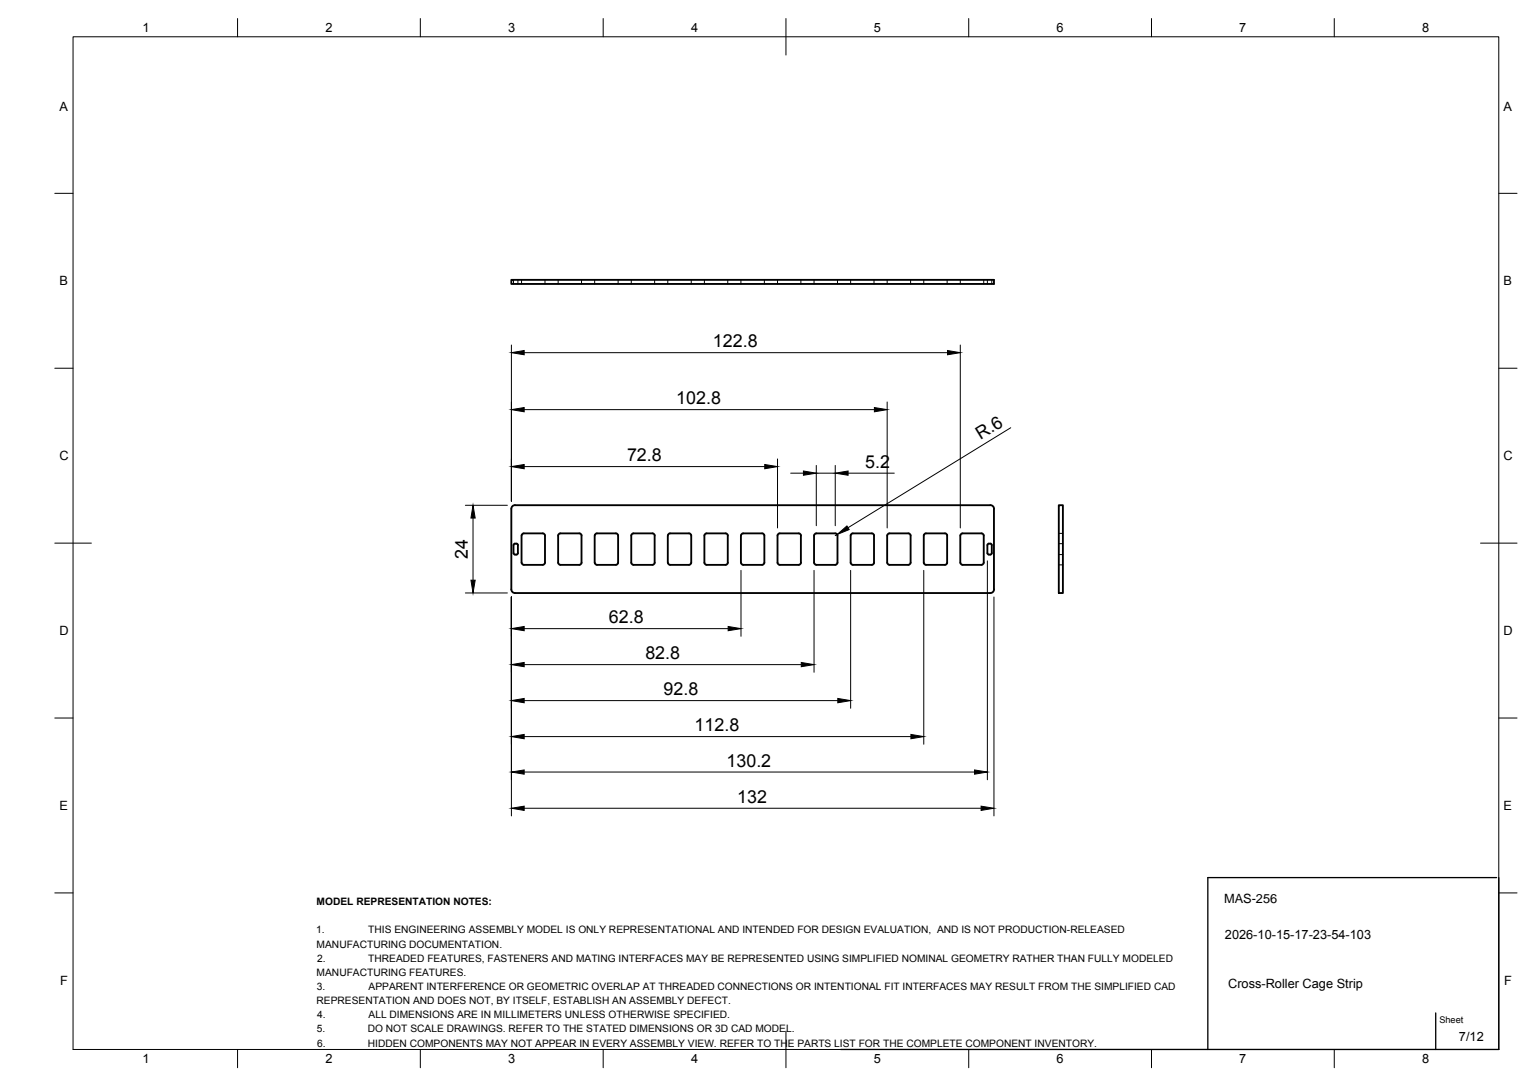
ISO-10303-21;
HEADER;
/* Generated by software containing ST-Developer
 * from STEP Tools, Inc. (www.steptools.com) 
 */

FILE_DESCRIPTION(
/* description */ (''),
/* implementation_level */ '2;1');

FILE_NAME(
/* name */ 'Cross-Roller Cage Strip.step',
/* time_stamp */ '2026-10-14T18:40:07-07:00',
/* author */ (''),
/* organization */ (''),
/* preprocessor_version */ 'ST-DEVELOPER v20.2',
/* originating_system */ 'Autodesk Translation Framework v15.15.0.0',
/* authorisation */ '');

FILE_SCHEMA (('AUTOMOTIVE_DESIGN { 1 0 10303 214 3 1 1 }'));
ENDSEC;

DATA;
#10=MECHANICAL_DESIGN_GEOMETRIC_PRESENTATION_REPRESENTATION('',(#835),#81040);
#815=SHAPE_REPRESENTATION_RELATIONSHIP('SRR','None',#81134,#825);
#825=ADVANCED_BREP_SHAPE_REPRESENTATION('',(#845),#81034);
#835=STYLED_ITEM('',(#81193),#845);
#845=MANIFOLD_SOLID_BREP('Body1',#15088);
#926=CYLINDRICAL_SURFACE('',#15818,0.400000000000027);
#927=CYLINDRICAL_SURFACE('',#15822,0.399999999999956);
#928=CYLINDRICAL_SURFACE('',#15826,0.399999999999945);
#929=CYLINDRICAL_SURFACE('',#15830,0.400000000000027);
#930=CYLINDRICAL_SURFACE('',#15834,0.399999999999996);
#931=CYLINDRICAL_SURFACE('',#15838,0.4);
#932=CYLINDRICAL_SURFACE('',#15842,0.399999999999996);
#933=CYLINDRICAL_SURFACE('',#15846,0.399999999999996);
#934=CYLINDRICAL_SURFACE('',#15850,0.600000000000005);
#935=CYLINDRICAL_SURFACE('',#15854,0.600000000000005);
#936=CYLINDRICAL_SURFACE('',#15858,0.600000000000005);
#937=CYLINDRICAL_SURFACE('',#15862,0.600000000000005);
#938=CYLINDRICAL_SURFACE('',#15866,0.600000000000005);
#939=CYLINDRICAL_SURFACE('',#15870,0.600000000000005);
#940=CYLINDRICAL_SURFACE('',#15874,0.600000000000005);
#941=CYLINDRICAL_SURFACE('',#15878,0.600000000000005);
#942=CYLINDRICAL_SURFACE('',#15882,0.599999999999987);
#943=CYLINDRICAL_SURFACE('',#15886,0.599999999999987);
#944=CYLINDRICAL_SURFACE('',#15890,0.599999999999987);
#945=CYLINDRICAL_SURFACE('',#15894,0.599999999999987);
#946=CYLINDRICAL_SURFACE('',#15898,0.599999999999987);
#947=CYLINDRICAL_SURFACE('',#15902,0.599999999999987);
#948=CYLINDRICAL_SURFACE('',#15906,0.599999999999987);
#949=CYLINDRICAL_SURFACE('',#15910,0.599999999999987);
#950=CYLINDRICAL_SURFACE('',#15914,0.599999999999987);
#951=CYLINDRICAL_SURFACE('',#15918,0.599999999999987);
#952=CYLINDRICAL_SURFACE('',#15922,0.599999999999987);
#953=CYLINDRICAL_SURFACE('',#15926,0.599999999999987);
#954=CYLINDRICAL_SURFACE('',#15930,0.600000000000001);
#955=CYLINDRICAL_SURFACE('',#15934,0.600000000000005);
#956=CYLINDRICAL_SURFACE('',#15938,0.599999999999998);
#957=CYLINDRICAL_SURFACE('',#15942,0.600000000000005);
#958=CYLINDRICAL_SURFACE('',#15946,0.600000000000001);
#959=CYLINDRICAL_SURFACE('',#15950,0.600000000000005);
#960=CYLINDRICAL_SURFACE('',#15954,0.600000000000003);
#961=CYLINDRICAL_SURFACE('',#15958,0.600000000000005);
#962=CYLINDRICAL_SURFACE('',#15962,0.599999999999996);
#963=CYLINDRICAL_SURFACE('',#15966,0.600000000000005);
#964=CYLINDRICAL_SURFACE('',#15970,0.599999999999998);
#965=CYLINDRICAL_SURFACE('',#15974,0.600000000000005);
#966=CYLINDRICAL_SURFACE('',#15978,0.599999999999987);
#967=CYLINDRICAL_SURFACE('',#15982,0.599999999999987);
#968=CYLINDRICAL_SURFACE('',#15986,0.599999999999987);
#969=CYLINDRICAL_SURFACE('',#15990,0.599999999999987);
#970=CYLINDRICAL_SURFACE('',#15994,0.600000000000001);
#971=CYLINDRICAL_SURFACE('',#15998,0.600000000000005);
#972=CYLINDRICAL_SURFACE('',#16002,0.600000000000003);
#973=CYLINDRICAL_SURFACE('',#16006,0.600000000000005);
#974=CYLINDRICAL_SURFACE('',#16010,0.599999999999987);
#975=CYLINDRICAL_SURFACE('',#16014,0.600000000000005);
#976=CYLINDRICAL_SURFACE('',#16018,0.600000000000005);
#977=CYLINDRICAL_SURFACE('',#16022,0.599999999999987);
#978=CYLINDRICAL_SURFACE('',#16026,0.600000000000005);
#979=CYLINDRICAL_SURFACE('',#16030,0.600000000000005);
#980=CYLINDRICAL_SURFACE('',#16034,0.600000000000005);
#981=CYLINDRICAL_SURFACE('',#16038,0.600000000000005);
#982=CYLINDRICAL_SURFACE('',#16042,0.600000000000027);
#983=CYLINDRICAL_SURFACE('',#16046,0.600000000000023);
#984=CYLINDRICAL_SURFACE('',#16050,0.600000000000025);
#985=CYLINDRICAL_SURFACE('',#16054,0.600000000000023);
#986=CYLINDRICAL_SURFACE('',#16058,1.);
#987=CYLINDRICAL_SURFACE('',#16062,1.00000000000001);
#988=CYLINDRICAL_SURFACE('',#16066,1.00000000000001);
#989=CYLINDRICAL_SURFACE('',#16070,1.);
#1176=FACE_BOUND('',#2884,.T.);
#1177=FACE_BOUND('',#2885,.T.);
#1178=FACE_BOUND('',#2886,.T.);
#1179=FACE_BOUND('',#2887,.T.);
#1180=FACE_BOUND('',#2888,.T.);
#1181=FACE_BOUND('',#2889,.T.);
#1182=FACE_BOUND('',#2890,.T.);
#1183=FACE_BOUND('',#2891,.T.);
#1184=FACE_BOUND('',#2892,.T.);
#1185=FACE_BOUND('',#2893,.T.);
#1186=FACE_BOUND('',#2894,.T.);
#1187=FACE_BOUND('',#2895,.T.);
#1188=FACE_BOUND('',#2896,.T.);
#1189=FACE_BOUND('',#2897,.T.);
#1190=FACE_BOUND('',#2898,.T.);
#1191=FACE_BOUND('',#2900,.T.);
#1192=FACE_BOUND('',#2901,.T.);
#1193=FACE_BOUND('',#2902,.T.);
#1194=FACE_BOUND('',#2903,.T.);
#1195=FACE_BOUND('',#2904,.T.);
#1196=FACE_BOUND('',#2905,.T.);
#1197=FACE_BOUND('',#2906,.T.);
#1198=FACE_BOUND('',#2907,.T.);
#1199=FACE_BOUND('',#2908,.T.);
#1200=FACE_BOUND('',#2909,.T.);
#1201=FACE_BOUND('',#2910,.T.);
#1202=FACE_BOUND('',#2911,.T.);
#1203=FACE_BOUND('',#2912,.T.);
#1204=FACE_BOUND('',#2913,.T.);
#1205=FACE_BOUND('',#2914,.T.);
#1362=PLANE('',#15817);
#1363=PLANE('',#15821);
#1364=PLANE('',#15825);
#1365=PLANE('',#15829);
#1366=PLANE('',#15833);
#1367=PLANE('',#15837);
#1368=PLANE('',#15841);
#1369=PLANE('',#15845);
#1370=PLANE('',#15849);
#1371=PLANE('',#15853);
#1372=PLANE('',#15857);
#1373=PLANE('',#15861);
#1374=PLANE('',#15865);
#1375=PLANE('',#15869);
#1376=PLANE('',#15873);
#1377=PLANE('',#15877);
#1378=PLANE('',#15881);
#1379=PLANE('',#15885);
#1380=PLANE('',#15889);
#1381=PLANE('',#15893);
#1382=PLANE('',#15897);
#1383=PLANE('',#15901);
#1384=PLANE('',#15905);
#1385=PLANE('',#15909);
#1386=PLANE('',#15913);
#1387=PLANE('',#15917);
#1388=PLANE('',#15921);
#1389=PLANE('',#15925);
#1390=PLANE('',#15929);
#1391=PLANE('',#15933);
#1392=PLANE('',#15937);
#1393=PLANE('',#15941);
#1394=PLANE('',#15945);
#1395=PLANE('',#15949);
#1396=PLANE('',#15953);
#1397=PLANE('',#15957);
#1398=PLANE('',#15961);
#1399=PLANE('',#15965);
#1400=PLANE('',#15969);
#1401=PLANE('',#15973);
#1402=PLANE('',#15977);
#1403=PLANE('',#15981);
#1404=PLANE('',#15985);
#1405=PLANE('',#15989);
#1406=PLANE('',#15993);
#1407=PLANE('',#15997);
#1408=PLANE('',#16001);
#1409=PLANE('',#16005);
#1410=PLANE('',#16009);
#1411=PLANE('',#16013);
#1412=PLANE('',#16017);
#1413=PLANE('',#16021);
#1414=PLANE('',#16025);
#1415=PLANE('',#16029);
#1416=PLANE('',#16033);
#1417=PLANE('',#16037);
#1418=PLANE('',#16041);
#1419=PLANE('',#16045);
#1420=PLANE('',#16049);
#1421=PLANE('',#16053);
#1422=PLANE('',#16057);
#1423=PLANE('',#16061);
#1424=PLANE('',#16065);
#1425=PLANE('',#16069);
#1426=PLANE('',#16073);
#1427=PLANE('',#16074);
#1919=FACE_OUTER_BOUND('',#2755,.T.);
#1920=FACE_OUTER_BOUND('',#2756,.T.);
#1921=FACE_OUTER_BOUND('',#2757,.T.);
#1922=FACE_OUTER_BOUND('',#2758,.T.);
#1923=FACE_OUTER_BOUND('',#2759,.T.);
#1924=FACE_OUTER_BOUND('',#2760,.T.);
#1925=FACE_OUTER_BOUND('',#2761,.T.);
#1926=FACE_OUTER_BOUND('',#2762,.T.);
#1927=FACE_OUTER_BOUND('',#2763,.T.);
#1928=FACE_OUTER_BOUND('',#2764,.T.);
#1929=FACE_OUTER_BOUND('',#2765,.T.);
#1930=FACE_OUTER_BOUND('',#2766,.T.);
#1931=FACE_OUTER_BOUND('',#2767,.T.);
#1932=FACE_OUTER_BOUND('',#2768,.T.);
#1933=FACE_OUTER_BOUND('',#2769,.T.);
#1934=FACE_OUTER_BOUND('',#2770,.T.);
#1935=FACE_OUTER_BOUND('',#2771,.T.);
#1936=FACE_OUTER_BOUND('',#2772,.T.);
#1937=FACE_OUTER_BOUND('',#2773,.T.);
#1938=FACE_OUTER_BOUND('',#2774,.T.);
#1939=FACE_OUTER_BOUND('',#2775,.T.);
#1940=FACE_OUTER_BOUND('',#2776,.T.);
#1941=FACE_OUTER_BOUND('',#2777,.T.);
#1942=FACE_OUTER_BOUND('',#2778,.T.);
#1943=FACE_OUTER_BOUND('',#2779,.T.);
#1944=FACE_OUTER_BOUND('',#2780,.T.);
#1945=FACE_OUTER_BOUND('',#2781,.T.);
#1946=FACE_OUTER_BOUND('',#2782,.T.);
#1947=FACE_OUTER_BOUND('',#2783,.T.);
#1948=FACE_OUTER_BOUND('',#2784,.T.);
#1949=FACE_OUTER_BOUND('',#2785,.T.);
#1950=FACE_OUTER_BOUND('',#2786,.T.);
#1951=FACE_OUTER_BOUND('',#2787,.T.);
#1952=FACE_OUTER_BOUND('',#2788,.T.);
#1953=FACE_OUTER_BOUND('',#2789,.T.);
#1954=FACE_OUTER_BOUND('',#2790,.T.);
#1955=FACE_OUTER_BOUND('',#2791,.T.);
#1956=FACE_OUTER_BOUND('',#2792,.T.);
#1957=FACE_OUTER_BOUND('',#2793,.T.);
#1958=FACE_OUTER_BOUND('',#2794,.T.);
#1959=FACE_OUTER_BOUND('',#2795,.T.);
#1960=FACE_OUTER_BOUND('',#2796,.T.);
#1961=FACE_OUTER_BOUND('',#2797,.T.);
#1962=FACE_OUTER_BOUND('',#2798,.T.);
#1963=FACE_OUTER_BOUND('',#2799,.T.);
#1964=FACE_OUTER_BOUND('',#2800,.T.);
#1965=FACE_OUTER_BOUND('',#2801,.T.);
#1966=FACE_OUTER_BOUND('',#2802,.T.);
#1967=FACE_OUTER_BOUND('',#2803,.T.);
#1968=FACE_OUTER_BOUND('',#2804,.T.);
#1969=FACE_OUTER_BOUND('',#2805,.T.);
#1970=FACE_OUTER_BOUND('',#2806,.T.);
#1971=FACE_OUTER_BOUND('',#2807,.T.);
#1972=FACE_OUTER_BOUND('',#2808,.T.);
#1973=FACE_OUTER_BOUND('',#2809,.T.);
#1974=FACE_OUTER_BOUND('',#2810,.T.);
#1975=FACE_OUTER_BOUND('',#2811,.T.);
#1976=FACE_OUTER_BOUND('',#2812,.T.);
#1977=FACE_OUTER_BOUND('',#2813,.T.);
#1978=FACE_OUTER_BOUND('',#2814,.T.);
#1979=FACE_OUTER_BOUND('',#2815,.T.);
#1980=FACE_OUTER_BOUND('',#2816,.T.);
#1981=FACE_OUTER_BOUND('',#2817,.T.);
#1982=FACE_OUTER_BOUND('',#2818,.T.);
#1983=FACE_OUTER_BOUND('',#2819,.T.);
#1984=FACE_OUTER_BOUND('',#2820,.T.);
#1985=FACE_OUTER_BOUND('',#2821,.T.);
#1986=FACE_OUTER_BOUND('',#2822,.T.);
#1987=FACE_OUTER_BOUND('',#2823,.T.);
#1988=FACE_OUTER_BOUND('',#2824,.T.);
#1989=FACE_OUTER_BOUND('',#2825,.T.);
#1990=FACE_OUTER_BOUND('',#2826,.T.);
#1991=FACE_OUTER_BOUND('',#2827,.T.);
#1992=FACE_OUTER_BOUND('',#2828,.T.);
#1993=FACE_OUTER_BOUND('',#2829,.T.);
#1994=FACE_OUTER_BOUND('',#2830,.T.);
#1995=FACE_OUTER_BOUND('',#2831,.T.);
#1996=FACE_OUTER_BOUND('',#2832,.T.);
#1997=FACE_OUTER_BOUND('',#2833,.T.);
#1998=FACE_OUTER_BOUND('',#2834,.T.);
#1999=FACE_OUTER_BOUND('',#2835,.T.);
#2000=FACE_OUTER_BOUND('',#2836,.T.);
#2001=FACE_OUTER_BOUND('',#2837,.T.);
#2002=FACE_OUTER_BOUND('',#2838,.T.);
#2003=FACE_OUTER_BOUND('',#2839,.T.);
#2004=FACE_OUTER_BOUND('',#2840,.T.);
#2005=FACE_OUTER_BOUND('',#2841,.T.);
#2006=FACE_OUTER_BOUND('',#2842,.T.);
#2007=FACE_OUTER_BOUND('',#2843,.T.);
#2008=FACE_OUTER_BOUND('',#2844,.T.);
#2009=FACE_OUTER_BOUND('',#2845,.T.);
#2010=FACE_OUTER_BOUND('',#2846,.T.);
#2011=FACE_OUTER_BOUND('',#2847,.T.);
#2012=FACE_OUTER_BOUND('',#2848,.T.);
#2013=FACE_OUTER_BOUND('',#2849,.T.);
#2014=FACE_OUTER_BOUND('',#2850,.T.);
#2015=FACE_OUTER_BOUND('',#2851,.T.);
#2016=FACE_OUTER_BOUND('',#2852,.T.);
#2017=FACE_OUTER_BOUND('',#2853,.T.);
#2018=FACE_OUTER_BOUND('',#2854,.T.);
#2019=FACE_OUTER_BOUND('',#2855,.T.);
#2020=FACE_OUTER_BOUND('',#2856,.T.);
#2021=FACE_OUTER_BOUND('',#2857,.T.);
#2022=FACE_OUTER_BOUND('',#2858,.T.);
#2023=FACE_OUTER_BOUND('',#2859,.T.);
#2024=FACE_OUTER_BOUND('',#2860,.T.);
#2025=FACE_OUTER_BOUND('',#2861,.T.);
#2026=FACE_OUTER_BOUND('',#2862,.T.);
#2027=FACE_OUTER_BOUND('',#2863,.T.);
#2028=FACE_OUTER_BOUND('',#2864,.T.);
#2029=FACE_OUTER_BOUND('',#2865,.T.);
#2030=FACE_OUTER_BOUND('',#2866,.T.);
#2031=FACE_OUTER_BOUND('',#2867,.T.);
#2032=FACE_OUTER_BOUND('',#2868,.T.);
#2033=FACE_OUTER_BOUND('',#2869,.T.);
#2034=FACE_OUTER_BOUND('',#2870,.T.);
#2035=FACE_OUTER_BOUND('',#2871,.T.);
#2036=FACE_OUTER_BOUND('',#2872,.T.);
#2037=FACE_OUTER_BOUND('',#2873,.T.);
#2038=FACE_OUTER_BOUND('',#2874,.T.);
#2039=FACE_OUTER_BOUND('',#2875,.T.);
#2040=FACE_OUTER_BOUND('',#2876,.T.);
#2041=FACE_OUTER_BOUND('',#2877,.T.);
#2042=FACE_OUTER_BOUND('',#2878,.T.);
#2043=FACE_OUTER_BOUND('',#2879,.T.);
#2044=FACE_OUTER_BOUND('',#2880,.T.);
#2045=FACE_OUTER_BOUND('',#2881,.T.);
#2046=FACE_OUTER_BOUND('',#2882,.T.);
#2047=FACE_OUTER_BOUND('',#2883,.T.);
#2048=FACE_OUTER_BOUND('',#2899,.T.);
#2755=EDGE_LOOP('',(#11400,#11401,#11402,#11403));
#2756=EDGE_LOOP('',(#11404,#11405,#11406,#11407));
#2757=EDGE_LOOP('',(#11408,#11409,#11410,#11411));
#2758=EDGE_LOOP('',(#11412,#11413,#11414,#11415));
#2759=EDGE_LOOP('',(#11416,#11417,#11418,#11419));
#2760=EDGE_LOOP('',(#11420,#11421,#11422,#11423));
#2761=EDGE_LOOP('',(#11424,#11425,#11426,#11427));
#2762=EDGE_LOOP('',(#11428,#11429,#11430,#11431));
#2763=EDGE_LOOP('',(#11432,#11433,#11434,#11435));
#2764=EDGE_LOOP('',(#11436,#11437,#11438,#11439));
#2765=EDGE_LOOP('',(#11440,#11441,#11442,#11443));
#2766=EDGE_LOOP('',(#11444,#11445,#11446,#11447));
#2767=EDGE_LOOP('',(#11448,#11449,#11450,#11451));
#2768=EDGE_LOOP('',(#11452,#11453,#11454,#11455));
#2769=EDGE_LOOP('',(#11456,#11457,#11458,#11459));
#2770=EDGE_LOOP('',(#11460,#11461,#11462,#11463));
#2771=EDGE_LOOP('',(#11464,#11465,#11466,#11467));
#2772=EDGE_LOOP('',(#11468,#11469,#11470,#11471));
#2773=EDGE_LOOP('',(#11472,#11473,#11474,#11475));
#2774=EDGE_LOOP('',(#11476,#11477,#11478,#11479));
#2775=EDGE_LOOP('',(#11480,#11481,#11482,#11483));
#2776=EDGE_LOOP('',(#11484,#11485,#11486,#11487));
#2777=EDGE_LOOP('',(#11488,#11489,#11490,#11491));
#2778=EDGE_LOOP('',(#11492,#11493,#11494,#11495));
#2779=EDGE_LOOP('',(#11496,#11497,#11498,#11499));
#2780=EDGE_LOOP('',(#11500,#11501,#11502,#11503));
#2781=EDGE_LOOP('',(#11504,#11505,#11506,#11507));
#2782=EDGE_LOOP('',(#11508,#11509,#11510,#11511));
#2783=EDGE_LOOP('',(#11512,#11513,#11514,#11515));
#2784=EDGE_LOOP('',(#11516,#11517,#11518,#11519));
#2785=EDGE_LOOP('',(#11520,#11521,#11522,#11523));
#2786=EDGE_LOOP('',(#11524,#11525,#11526,#11527));
#2787=EDGE_LOOP('',(#11528,#11529,#11530,#11531));
#2788=EDGE_LOOP('',(#11532,#11533,#11534,#11535));
#2789=EDGE_LOOP('',(#11536,#11537,#11538,#11539));
#2790=EDGE_LOOP('',(#11540,#11541,#11542,#11543));
#2791=EDGE_LOOP('',(#11544,#11545,#11546,#11547));
#2792=EDGE_LOOP('',(#11548,#11549,#11550,#11551));
#2793=EDGE_LOOP('',(#11552,#11553,#11554,#11555));
#2794=EDGE_LOOP('',(#11556,#11557,#11558,#11559));
#2795=EDGE_LOOP('',(#11560,#11561,#11562,#11563));
#2796=EDGE_LOOP('',(#11564,#11565,#11566,#11567));
#2797=EDGE_LOOP('',(#11568,#11569,#11570,#11571));
#2798=EDGE_LOOP('',(#11572,#11573,#11574,#11575));
#2799=EDGE_LOOP('',(#11576,#11577,#11578,#11579));
#2800=EDGE_LOOP('',(#11580,#11581,#11582,#11583));
#2801=EDGE_LOOP('',(#11584,#11585,#11586,#11587));
#2802=EDGE_LOOP('',(#11588,#11589,#11590,#11591));
#2803=EDGE_LOOP('',(#11592,#11593,#11594,#11595));
#2804=EDGE_LOOP('',(#11596,#11597,#11598,#11599));
#2805=EDGE_LOOP('',(#11600,#11601,#11602,#11603));
#2806=EDGE_LOOP('',(#11604,#11605,#11606,#11607));
#2807=EDGE_LOOP('',(#11608,#11609,#11610,#11611));
#2808=EDGE_LOOP('',(#11612,#11613,#11614,#11615));
#2809=EDGE_LOOP('',(#11616,#11617,#11618,#11619));
#2810=EDGE_LOOP('',(#11620,#11621,#11622,#11623));
#2811=EDGE_LOOP('',(#11624,#11625,#11626,#11627));
#2812=EDGE_LOOP('',(#11628,#11629,#11630,#11631));
#2813=EDGE_LOOP('',(#11632,#11633,#11634,#11635));
#2814=EDGE_LOOP('',(#11636,#11637,#11638,#11639));
#2815=EDGE_LOOP('',(#11640,#11641,#11642,#11643));
#2816=EDGE_LOOP('',(#11644,#11645,#11646,#11647));
#2817=EDGE_LOOP('',(#11648,#11649,#11650,#11651));
#2818=EDGE_LOOP('',(#11652,#11653,#11654,#11655));
#2819=EDGE_LOOP('',(#11656,#11657,#11658,#11659));
#2820=EDGE_LOOP('',(#11660,#11661,#11662,#11663));
#2821=EDGE_LOOP('',(#11664,#11665,#11666,#11667));
#2822=EDGE_LOOP('',(#11668,#11669,#11670,#11671));
#2823=EDGE_LOOP('',(#11672,#11673,#11674,#11675));
#2824=EDGE_LOOP('',(#11676,#11677,#11678,#11679));
#2825=EDGE_LOOP('',(#11680,#11681,#11682,#11683));
#2826=EDGE_LOOP('',(#11684,#11685,#11686,#11687));
#2827=EDGE_LOOP('',(#11688,#11689,#11690,#11691));
#2828=EDGE_LOOP('',(#11692,#11693,#11694,#11695));
#2829=EDGE_LOOP('',(#11696,#11697,#11698,#11699));
#2830=EDGE_LOOP('',(#11700,#11701,#11702,#11703));
#2831=EDGE_LOOP('',(#11704,#11705,#11706,#11707));
#2832=EDGE_LOOP('',(#11708,#11709,#11710,#11711));
#2833=EDGE_LOOP('',(#11712,#11713,#11714,#11715));
#2834=EDGE_LOOP('',(#11716,#11717,#11718,#11719));
#2835=EDGE_LOOP('',(#11720,#11721,#11722,#11723));
#2836=EDGE_LOOP('',(#11724,#11725,#11726,#11727));
#2837=EDGE_LOOP('',(#11728,#11729,#11730,#11731));
#2838=EDGE_LOOP('',(#11732,#11733,#11734,#11735));
#2839=EDGE_LOOP('',(#11736,#11737,#11738,#11739));
#2840=EDGE_LOOP('',(#11740,#11741,#11742,#11743));
#2841=EDGE_LOOP('',(#11744,#11745,#11746,#11747));
#2842=EDGE_LOOP('',(#11748,#11749,#11750,#11751));
#2843=EDGE_LOOP('',(#11752,#11753,#11754,#11755));
#2844=EDGE_LOOP('',(#11756,#11757,#11758,#11759));
#2845=EDGE_LOOP('',(#11760,#11761,#11762,#11763));
#2846=EDGE_LOOP('',(#11764,#11765,#11766,#11767));
#2847=EDGE_LOOP('',(#11768,#11769,#11770,#11771));
#2848=EDGE_LOOP('',(#11772,#11773,#11774,#11775));
#2849=EDGE_LOOP('',(#11776,#11777,#11778,#11779));
#2850=EDGE_LOOP('',(#11780,#11781,#11782,#11783));
#2851=EDGE_LOOP('',(#11784,#11785,#11786,#11787));
#2852=EDGE_LOOP('',(#11788,#11789,#11790,#11791));
#2853=EDGE_LOOP('',(#11792,#11793,#11794,#11795));
#2854=EDGE_LOOP('',(#11796,#11797,#11798,#11799));
#2855=EDGE_LOOP('',(#11800,#11801,#11802,#11803));
#2856=EDGE_LOOP('',(#11804,#11805,#11806,#11807));
#2857=EDGE_LOOP('',(#11808,#11809,#11810,#11811));
#2858=EDGE_LOOP('',(#11812,#11813,#11814,#11815));
#2859=EDGE_LOOP('',(#11816,#11817,#11818,#11819));
#2860=EDGE_LOOP('',(#11820,#11821,#11822,#11823));
#2861=EDGE_LOOP('',(#11824,#11825,#11826,#11827));
#2862=EDGE_LOOP('',(#11828,#11829,#11830,#11831));
#2863=EDGE_LOOP('',(#11832,#11833,#11834,#11835));
#2864=EDGE_LOOP('',(#11836,#11837,#11838,#11839));
#2865=EDGE_LOOP('',(#11840,#11841,#11842,#11843));
#2866=EDGE_LOOP('',(#11844,#11845,#11846,#11847));
#2867=EDGE_LOOP('',(#11848,#11849,#11850,#11851));
#2868=EDGE_LOOP('',(#11852,#11853,#11854,#11855));
#2869=EDGE_LOOP('',(#11856,#11857,#11858,#11859));
#2870=EDGE_LOOP('',(#11860,#11861,#11862,#11863));
#2871=EDGE_LOOP('',(#11864,#11865,#11866,#11867));
#2872=EDGE_LOOP('',(#11868,#11869,#11870,#11871));
#2873=EDGE_LOOP('',(#11872,#11873,#11874,#11875));
#2874=EDGE_LOOP('',(#11876,#11877,#11878,#11879));
#2875=EDGE_LOOP('',(#11880,#11881,#11882,#11883));
#2876=EDGE_LOOP('',(#11884,#11885,#11886,#11887));
#2877=EDGE_LOOP('',(#11888,#11889,#11890,#11891));
#2878=EDGE_LOOP('',(#11892,#11893,#11894,#11895));
#2879=EDGE_LOOP('',(#11896,#11897,#11898,#11899));
#2880=EDGE_LOOP('',(#11900,#11901,#11902,#11903));
#2881=EDGE_LOOP('',(#11904,#11905,#11906,#11907));
#2882=EDGE_LOOP('',(#11908,#11909,#11910,#11911));
#2883=EDGE_LOOP('',(#11912,#11913,#11914,#11915,#11916,#11917,#11918,#11919));
#2884=EDGE_LOOP('',(#11920,#11921,#11922,#11923,#11924,#11925,#11926,#11927));
#2885=EDGE_LOOP('',(#11928,#11929,#11930,#11931,#11932,#11933,#11934,#11935));
#2886=EDGE_LOOP('',(#11936,#11937,#11938,#11939,#11940,#11941,#11942,#11943));
#2887=EDGE_LOOP('',(#11944,#11945,#11946,#11947,#11948,#11949,#11950,#11951));
#2888=EDGE_LOOP('',(#11952,#11953,#11954,#11955,#11956,#11957,#11958,#11959));
#2889=EDGE_LOOP('',(#11960,#11961,#11962,#11963,#11964,#11965,#11966,#11967));
#2890=EDGE_LOOP('',(#11968,#11969,#11970,#11971,#11972,#11973,#11974,#11975));
#2891=EDGE_LOOP('',(#11976,#11977,#11978,#11979,#11980,#11981,#11982,#11983));
#2892=EDGE_LOOP('',(#11984,#11985,#11986,#11987,#11988,#11989,#11990,#11991));
#2893=EDGE_LOOP('',(#11992,#11993,#11994,#11995,#11996,#11997,#11998,#11999));
#2894=EDGE_LOOP('',(#12000,#12001,#12002,#12003,#12004,#12005,#12006,#12007));
#2895=EDGE_LOOP('',(#12008,#12009,#12010,#12011,#12012,#12013,#12014,#12015));
#2896=EDGE_LOOP('',(#12016,#12017,#12018,#12019,#12020,#12021,#12022,#12023));
#2897=EDGE_LOOP('',(#12024,#12025,#12026,#12027,#12028,#12029,#12030,#12031));
#2898=EDGE_LOOP('',(#12032,#12033,#12034,#12035,#12036,#12037,#12038,#12039));
#2899=EDGE_LOOP('',(#12040,#12041,#12042,#12043,#12044,#12045,#12046,#12047));
#2900=EDGE_LOOP('',(#12048,#12049,#12050,#12051,#12052,#12053,#12054,#12055));
#2901=EDGE_LOOP('',(#12056,#12057,#12058,#12059,#12060,#12061,#12062,#12063));
#2902=EDGE_LOOP('',(#12064,#12065,#12066,#12067,#12068,#12069,#12070,#12071));
#2903=EDGE_LOOP('',(#12072,#12073,#12074,#12075,#12076,#12077,#12078,#12079));
#2904=EDGE_LOOP('',(#12080,#12081,#12082,#12083,#12084,#12085,#12086,#12087));
#2905=EDGE_LOOP('',(#12088,#12089,#12090,#12091,#12092,#12093,#12094,#12095));
#2906=EDGE_LOOP('',(#12096,#12097,#12098,#12099,#12100,#12101,#12102,#12103));
#2907=EDGE_LOOP('',(#12104,#12105,#12106,#12107,#12108,#12109,#12110,#12111));
#2908=EDGE_LOOP('',(#12112,#12113,#12114,#12115,#12116,#12117,#12118,#12119));
#2909=EDGE_LOOP('',(#12120,#12121,#12122,#12123,#12124,#12125,#12126,#12127));
#2910=EDGE_LOOP('',(#12128,#12129,#12130,#12131,#12132,#12133,#12134,#12135));
#2911=EDGE_LOOP('',(#12136,#12137,#12138,#12139,#12140,#12141,#12142,#12143));
#2912=EDGE_LOOP('',(#12144,#12145,#12146,#12147,#12148,#12149,#12150,#12151));
#2913=EDGE_LOOP('',(#12152,#12153,#12154,#12155,#12156,#12157,#12158,#12159));
#2914=EDGE_LOOP('',(#12160,#12161,#12162,#12163,#12164,#12165,#12166,#12167));
#3730=LINE('',#22250,#4842);
#3731=LINE('',#22252,#4843);
#3732=LINE('',#22254,#4844);
#3733=LINE('',#22255,#4845);
#3734=LINE('',#22260,#4846);
#3735=LINE('',#22264,#4847);
#3736=LINE('',#22266,#4848);
#3737=LINE('',#22267,#4849);
#3738=LINE('',#22272,#4850);
#3739=LINE('',#22276,#4851);
#3740=LINE('',#22278,#4852);
#3741=LINE('',#22279,#4853);
#3742=LINE('',#22284,#4854);
#3743=LINE('',#22288,#4855);
#3744=LINE('',#22290,#4856);
#3745=LINE('',#22291,#4857);
#3746=LINE('',#22298,#4858);
#3747=LINE('',#22300,#4859);
#3748=LINE('',#22302,#4860);
#3749=LINE('',#22303,#4861);
#3750=LINE('',#22308,#4862);
#3751=LINE('',#22312,#4863);
#3752=LINE('',#22314,#4864);
#3753=LINE('',#22315,#4865);
#3754=LINE('',#22320,#4866);
#3755=LINE('',#22324,#4867);
#3756=LINE('',#22326,#4868);
#3757=LINE('',#22327,#4869);
#3758=LINE('',#22332,#4870);
#3759=LINE('',#22336,#4871);
#3760=LINE('',#22338,#4872);
#3761=LINE('',#22339,#4873);
#3762=LINE('',#22346,#4874);
#3763=LINE('',#22348,#4875);
#3764=LINE('',#22350,#4876);
#3765=LINE('',#22351,#4877);
#3766=LINE('',#22356,#4878);
#3767=LINE('',#22360,#4879);
#3768=LINE('',#22362,#4880);
#3769=LINE('',#22363,#4881);
#3770=LINE('',#22368,#4882);
#3771=LINE('',#22372,#4883);
#3772=LINE('',#22374,#4884);
#3773=LINE('',#22375,#4885);
#3774=LINE('',#22380,#4886);
#3775=LINE('',#22384,#4887);
#3776=LINE('',#22386,#4888);
#3777=LINE('',#22387,#4889);
#3778=LINE('',#22394,#4890);
#3779=LINE('',#22396,#4891);
#3780=LINE('',#22398,#4892);
#3781=LINE('',#22399,#4893);
#3782=LINE('',#22404,#4894);
#3783=LINE('',#22408,#4895);
#3784=LINE('',#22410,#4896);
#3785=LINE('',#22411,#4897);
#3786=LINE('',#22416,#4898);
#3787=LINE('',#22420,#4899);
#3788=LINE('',#22422,#4900);
#3789=LINE('',#22423,#4901);
#3790=LINE('',#22428,#4902);
#3791=LINE('',#22432,#4903);
#3792=LINE('',#22434,#4904);
#3793=LINE('',#22435,#4905);
#3794=LINE('',#22442,#4906);
#3795=LINE('',#22444,#4907);
#3796=LINE('',#22446,#4908);
#3797=LINE('',#22447,#4909);
#3798=LINE('',#22452,#4910);
#3799=LINE('',#22456,#4911);
#3800=LINE('',#22458,#4912);
#3801=LINE('',#22459,#4913);
#3802=LINE('',#22464,#4914);
#3803=LINE('',#22468,#4915);
#3804=LINE('',#22470,#4916);
#3805=LINE('',#22471,#4917);
#3806=LINE('',#22476,#4918);
#3807=LINE('',#22480,#4919);
#3808=LINE('',#22482,#4920);
#3809=LINE('',#22483,#4921);
#3810=LINE('',#22490,#4922);
#3811=LINE('',#22492,#4923);
#3812=LINE('',#22494,#4924);
#3813=LINE('',#22495,#4925);
#3814=LINE('',#22500,#4926);
#3815=LINE('',#22504,#4927);
#3816=LINE('',#22506,#4928);
#3817=LINE('',#22507,#4929);
#3818=LINE('',#22512,#4930);
#3819=LINE('',#22516,#4931);
#3820=LINE('',#22518,#4932);
#3821=LINE('',#22519,#4933);
#3822=LINE('',#22524,#4934);
#3823=LINE('',#22528,#4935);
#3824=LINE('',#22530,#4936);
#3825=LINE('',#22531,#4937);
#3826=LINE('',#22538,#4938);
#3827=LINE('',#22540,#4939);
#3828=LINE('',#22542,#4940);
#3829=LINE('',#22543,#4941);
#3830=LINE('',#22548,#4942);
#3831=LINE('',#22552,#4943);
#3832=LINE('',#22554,#4944);
#3833=LINE('',#22555,#4945);
#3834=LINE('',#22560,#4946);
#3835=LINE('',#22564,#4947);
#3836=LINE('',#22566,#4948);
#3837=LINE('',#22567,#4949);
#3838=LINE('',#22572,#4950);
#3839=LINE('',#22576,#4951);
#3840=LINE('',#22578,#4952);
#3841=LINE('',#22579,#4953);
#3842=LINE('',#22586,#4954);
#3843=LINE('',#22588,#4955);
#3844=LINE('',#22590,#4956);
#3845=LINE('',#22591,#4957);
#3846=LINE('',#22596,#4958);
#3847=LINE('',#22600,#4959);
#3848=LINE('',#22602,#4960);
#3849=LINE('',#22603,#4961);
#3850=LINE('',#22608,#4962);
#3851=LINE('',#22612,#4963);
#3852=LINE('',#22614,#4964);
#3853=LINE('',#22615,#4965);
#3854=LINE('',#22620,#4966);
#3855=LINE('',#22624,#4967);
#3856=LINE('',#22626,#4968);
#3857=LINE('',#22627,#4969);
#3858=LINE('',#22634,#4970);
#3859=LINE('',#22636,#4971);
#3860=LINE('',#22638,#4972);
#3861=LINE('',#22639,#4973);
#3862=LINE('',#22644,#4974);
#3863=LINE('',#22648,#4975);
#3864=LINE('',#22650,#4976);
#3865=LINE('',#22651,#4977);
#3866=LINE('',#22656,#4978);
#3867=LINE('',#22660,#4979);
#3868=LINE('',#22662,#4980);
#3869=LINE('',#22663,#4981);
#3870=LINE('',#22668,#4982);
#3871=LINE('',#22672,#4983);
#3872=LINE('',#22674,#4984);
#3873=LINE('',#22675,#4985);
#3874=LINE('',#22682,#4986);
#3875=LINE('',#22684,#4987);
#3876=LINE('',#22686,#4988);
#3877=LINE('',#22687,#4989);
#3878=LINE('',#22692,#4990);
#3879=LINE('',#22696,#4991);
#3880=LINE('',#22698,#4992);
#3881=LINE('',#22699,#4993);
#3882=LINE('',#22704,#4994);
#3883=LINE('',#22708,#4995);
#3884=LINE('',#22710,#4996);
#3885=LINE('',#22711,#4997);
#3886=LINE('',#22716,#4998);
#3887=LINE('',#22720,#4999);
#3888=LINE('',#22722,#5000);
#3889=LINE('',#22723,#5001);
#3890=LINE('',#22730,#5002);
#3891=LINE('',#22732,#5003);
#3892=LINE('',#22734,#5004);
#3893=LINE('',#22735,#5005);
#3894=LINE('',#22740,#5006);
#3895=LINE('',#22744,#5007);
#3896=LINE('',#22746,#5008);
#3897=LINE('',#22747,#5009);
#3898=LINE('',#22752,#5010);
#3899=LINE('',#22756,#5011);
#3900=LINE('',#22758,#5012);
#3901=LINE('',#22759,#5013);
#3902=LINE('',#22764,#5014);
#3903=LINE('',#22768,#5015);
#3904=LINE('',#22770,#5016);
#3905=LINE('',#22771,#5017);
#3906=LINE('',#22778,#5018);
#3907=LINE('',#22780,#5019);
#3908=LINE('',#22782,#5020);
#3909=LINE('',#22783,#5021);
#3910=LINE('',#22788,#5022);
#3911=LINE('',#22792,#5023);
#3912=LINE('',#22794,#5024);
#3913=LINE('',#22795,#5025);
#3914=LINE('',#22800,#5026);
#3915=LINE('',#22804,#5027);
#3916=LINE('',#22806,#5028);
#3917=LINE('',#22807,#5029);
#3918=LINE('',#22812,#5030);
#3919=LINE('',#22816,#5031);
#3920=LINE('',#22818,#5032);
#3921=LINE('',#22819,#5033);
#3922=LINE('',#22826,#5034);
#3923=LINE('',#22828,#5035);
#3924=LINE('',#22830,#5036);
#3925=LINE('',#22831,#5037);
#3926=LINE('',#22836,#5038);
#3927=LINE('',#22840,#5039);
#3928=LINE('',#22842,#5040);
#3929=LINE('',#22843,#5041);
#3930=LINE('',#22848,#5042);
#3931=LINE('',#22852,#5043);
#3932=LINE('',#22854,#5044);
#3933=LINE('',#22855,#5045);
#3934=LINE('',#22860,#5046);
#3935=LINE('',#22864,#5047);
#3936=LINE('',#22866,#5048);
#3937=LINE('',#22867,#5049);
#3938=LINE('',#22874,#5050);
#3939=LINE('',#22876,#5051);
#3940=LINE('',#22878,#5052);
#3941=LINE('',#22879,#5053);
#3942=LINE('',#22884,#5054);
#3943=LINE('',#22888,#5055);
#3944=LINE('',#22890,#5056);
#3945=LINE('',#22891,#5057);
#3946=LINE('',#22896,#5058);
#3947=LINE('',#22900,#5059);
#3948=LINE('',#22902,#5060);
#3949=LINE('',#22903,#5061);
#3950=LINE('',#22908,#5062);
#3951=LINE('',#22912,#5063);
#3952=LINE('',#22914,#5064);
#3953=LINE('',#22915,#5065);
#3954=LINE('',#22922,#5066);
#3955=LINE('',#22924,#5067);
#3956=LINE('',#22926,#5068);
#3957=LINE('',#22927,#5069);
#3958=LINE('',#22932,#5070);
#3959=LINE('',#22936,#5071);
#3960=LINE('',#22938,#5072);
#3961=LINE('',#22939,#5073);
#3962=LINE('',#22944,#5074);
#3963=LINE('',#22948,#5075);
#3964=LINE('',#22950,#5076);
#3965=LINE('',#22951,#5077);
#3966=LINE('',#22956,#5078);
#3967=LINE('',#22960,#5079);
#3968=LINE('',#22962,#5080);
#3969=LINE('',#22963,#5081);
#3970=LINE('',#22970,#5082);
#3971=LINE('',#22972,#5083);
#3972=LINE('',#22974,#5084);
#3973=LINE('',#22975,#5085);
#3974=LINE('',#22981,#5086);
#3975=LINE('',#22984,#5087);
#3976=LINE('',#22986,#5088);
#3977=LINE('',#22987,#5089);
#3978=LINE('',#22993,#5090);
#3979=LINE('',#22996,#5091);
#3980=LINE('',#22998,#5092);
#3981=LINE('',#22999,#5093);
#3982=LINE('',#23005,#5094);
#3983=LINE('',#23008,#5095);
#3984=LINE('',#23010,#5096);
#3985=LINE('',#23011,#5097);
#4842=VECTOR('',#18356,10.);
#4843=VECTOR('',#18357,10.);
#4844=VECTOR('',#18358,10.);
#4845=VECTOR('',#18359,10.);
#4846=VECTOR('',#18364,10.);
#4847=VECTOR('',#18369,10.);
#4848=VECTOR('',#18370,10.);
#4849=VECTOR('',#18371,10.);
#4850=VECTOR('',#18376,10.);
#4851=VECTOR('',#18381,10.);
#4852=VECTOR('',#18382,10.);
#4853=VECTOR('',#18383,10.);
#4854=VECTOR('',#18388,10.);
#4855=VECTOR('',#18393,10.);
#4856=VECTOR('',#18394,10.);
#4857=VECTOR('',#18395,10.);
#4858=VECTOR('',#18404,10.);
#4859=VECTOR('',#18405,10.);
#4860=VECTOR('',#18406,10.);
#4861=VECTOR('',#18407,10.);
#4862=VECTOR('',#18412,10.);
#4863=VECTOR('',#18417,10.);
#4864=VECTOR('',#18418,10.);
#4865=VECTOR('',#18419,10.);
#4866=VECTOR('',#18424,10.);
#4867=VECTOR('',#18429,10.);
#4868=VECTOR('',#18430,10.);
#4869=VECTOR('',#18431,10.);
#4870=VECTOR('',#18436,10.);
#4871=VECTOR('',#18441,10.);
#4872=VECTOR('',#18442,10.);
#4873=VECTOR('',#18443,10.);
#4874=VECTOR('',#18452,10.);
#4875=VECTOR('',#18453,10.);
#4876=VECTOR('',#18454,10.);
#4877=VECTOR('',#18455,10.);
#4878=VECTOR('',#18460,10.);
#4879=VECTOR('',#18465,10.);
#4880=VECTOR('',#18466,10.);
#4881=VECTOR('',#18467,10.);
#4882=VECTOR('',#18472,10.);
#4883=VECTOR('',#18477,10.);
#4884=VECTOR('',#18478,10.);
#4885=VECTOR('',#18479,10.);
#4886=VECTOR('',#18484,10.);
#4887=VECTOR('',#18489,10.);
#4888=VECTOR('',#18490,10.);
#4889=VECTOR('',#18491,10.);
#4890=VECTOR('',#18500,10.);
#4891=VECTOR('',#18501,10.);
#4892=VECTOR('',#18502,10.);
#4893=VECTOR('',#18503,10.);
#4894=VECTOR('',#18508,10.);
#4895=VECTOR('',#18513,10.);
#4896=VECTOR('',#18514,10.);
#4897=VECTOR('',#18515,10.);
#4898=VECTOR('',#18520,10.);
#4899=VECTOR('',#18525,10.);
#4900=VECTOR('',#18526,10.);
#4901=VECTOR('',#18527,10.);
#4902=VECTOR('',#18532,10.);
#4903=VECTOR('',#18537,10.);
#4904=VECTOR('',#18538,10.);
#4905=VECTOR('',#18539,10.);
#4906=VECTOR('',#18548,10.);
#4907=VECTOR('',#18549,10.);
#4908=VECTOR('',#18550,10.);
#4909=VECTOR('',#18551,10.);
#4910=VECTOR('',#18556,10.);
#4911=VECTOR('',#18561,10.);
#4912=VECTOR('',#18562,10.);
#4913=VECTOR('',#18563,10.);
#4914=VECTOR('',#18568,10.);
#4915=VECTOR('',#18573,10.);
#4916=VECTOR('',#18574,10.);
#4917=VECTOR('',#18575,10.);
#4918=VECTOR('',#18580,10.);
#4919=VECTOR('',#18585,10.);
#4920=VECTOR('',#18586,10.);
#4921=VECTOR('',#18587,10.);
#4922=VECTOR('',#18596,10.);
#4923=VECTOR('',#18597,10.);
#4924=VECTOR('',#18598,10.);
#4925=VECTOR('',#18599,10.);
#4926=VECTOR('',#18604,10.);
#4927=VECTOR('',#18609,10.);
#4928=VECTOR('',#18610,10.);
#4929=VECTOR('',#18611,10.);
#4930=VECTOR('',#18616,10.);
#4931=VECTOR('',#18621,10.);
#4932=VECTOR('',#18622,10.);
#4933=VECTOR('',#18623,10.);
#4934=VECTOR('',#18628,10.);
#4935=VECTOR('',#18633,10.);
#4936=VECTOR('',#18634,10.);
#4937=VECTOR('',#18635,10.);
#4938=VECTOR('',#18644,10.);
#4939=VECTOR('',#18645,10.);
#4940=VECTOR('',#18646,10.);
#4941=VECTOR('',#18647,10.);
#4942=VECTOR('',#18652,10.);
#4943=VECTOR('',#18657,10.);
#4944=VECTOR('',#18658,10.);
#4945=VECTOR('',#18659,10.);
#4946=VECTOR('',#18664,10.);
#4947=VECTOR('',#18669,10.);
#4948=VECTOR('',#18670,10.);
#4949=VECTOR('',#18671,10.);
#4950=VECTOR('',#18676,10.);
#4951=VECTOR('',#18681,10.);
#4952=VECTOR('',#18682,10.);
#4953=VECTOR('',#18683,10.);
#4954=VECTOR('',#18692,10.);
#4955=VECTOR('',#18693,10.);
#4956=VECTOR('',#18694,10.);
#4957=VECTOR('',#18695,10.);
#4958=VECTOR('',#18700,10.);
#4959=VECTOR('',#18705,10.);
#4960=VECTOR('',#18706,10.);
#4961=VECTOR('',#18707,10.);
#4962=VECTOR('',#18712,10.);
#4963=VECTOR('',#18717,10.);
#4964=VECTOR('',#18718,10.);
#4965=VECTOR('',#18719,10.);
#4966=VECTOR('',#18724,10.);
#4967=VECTOR('',#18729,10.);
#4968=VECTOR('',#18730,10.);
#4969=VECTOR('',#18731,10.);
#4970=VECTOR('',#18740,10.);
#4971=VECTOR('',#18741,10.);
#4972=VECTOR('',#18742,10.);
#4973=VECTOR('',#18743,10.);
#4974=VECTOR('',#18748,10.);
#4975=VECTOR('',#18753,10.);
#4976=VECTOR('',#18754,10.);
#4977=VECTOR('',#18755,10.);
#4978=VECTOR('',#18760,10.);
#4979=VECTOR('',#18765,10.);
#4980=VECTOR('',#18766,10.);
#4981=VECTOR('',#18767,10.);
#4982=VECTOR('',#18772,10.);
#4983=VECTOR('',#18777,10.);
#4984=VECTOR('',#18778,10.);
#4985=VECTOR('',#18779,10.);
#4986=VECTOR('',#18788,10.);
#4987=VECTOR('',#18789,10.);
#4988=VECTOR('',#18790,10.);
#4989=VECTOR('',#18791,10.);
#4990=VECTOR('',#18796,10.);
#4991=VECTOR('',#18801,10.);
#4992=VECTOR('',#18802,10.);
#4993=VECTOR('',#18803,10.);
#4994=VECTOR('',#18808,10.);
#4995=VECTOR('',#18813,10.);
#4996=VECTOR('',#18814,10.);
#4997=VECTOR('',#18815,10.);
#4998=VECTOR('',#18820,10.);
#4999=VECTOR('',#18825,10.);
#5000=VECTOR('',#18826,10.);
#5001=VECTOR('',#18827,10.);
#5002=VECTOR('',#18836,10.);
#5003=VECTOR('',#18837,10.);
#5004=VECTOR('',#18838,10.);
#5005=VECTOR('',#18839,10.);
#5006=VECTOR('',#18844,10.);
#5007=VECTOR('',#18849,10.);
#5008=VECTOR('',#18850,10.);
#5009=VECTOR('',#18851,10.);
#5010=VECTOR('',#18856,10.);
#5011=VECTOR('',#18861,10.);
#5012=VECTOR('',#18862,10.);
#5013=VECTOR('',#18863,10.);
#5014=VECTOR('',#18868,10.);
#5015=VECTOR('',#18873,10.);
#5016=VECTOR('',#18874,10.);
#5017=VECTOR('',#18875,10.);
#5018=VECTOR('',#18884,10.);
#5019=VECTOR('',#18885,10.);
#5020=VECTOR('',#18886,10.);
#5021=VECTOR('',#18887,10.);
#5022=VECTOR('',#18892,10.);
#5023=VECTOR('',#18897,10.);
#5024=VECTOR('',#18898,10.);
#5025=VECTOR('',#18899,10.);
#5026=VECTOR('',#18904,10.);
#5027=VECTOR('',#18909,10.);
#5028=VECTOR('',#18910,10.);
#5029=VECTOR('',#18911,10.);
#5030=VECTOR('',#18916,10.);
#5031=VECTOR('',#18921,10.);
#5032=VECTOR('',#18922,10.);
#5033=VECTOR('',#18923,10.);
#5034=VECTOR('',#18932,10.);
#5035=VECTOR('',#18933,10.);
#5036=VECTOR('',#18934,10.);
#5037=VECTOR('',#18935,10.);
#5038=VECTOR('',#18940,10.);
#5039=VECTOR('',#18945,10.);
#5040=VECTOR('',#18946,10.);
#5041=VECTOR('',#18947,10.);
#5042=VECTOR('',#18952,10.);
#5043=VECTOR('',#18957,10.);
#5044=VECTOR('',#18958,10.);
#5045=VECTOR('',#18959,10.);
#5046=VECTOR('',#18964,10.);
#5047=VECTOR('',#18969,10.);
#5048=VECTOR('',#18970,10.);
#5049=VECTOR('',#18971,10.);
#5050=VECTOR('',#18980,10.);
#5051=VECTOR('',#18981,10.);
#5052=VECTOR('',#18982,10.);
#5053=VECTOR('',#18983,10.);
#5054=VECTOR('',#18988,10.);
#5055=VECTOR('',#18993,10.);
#5056=VECTOR('',#18994,10.);
#5057=VECTOR('',#18995,10.);
#5058=VECTOR('',#19000,10.);
#5059=VECTOR('',#19005,10.);
#5060=VECTOR('',#19006,10.);
#5061=VECTOR('',#19007,10.);
#5062=VECTOR('',#19012,10.);
#5063=VECTOR('',#19017,10.);
#5064=VECTOR('',#19018,10.);
#5065=VECTOR('',#19019,10.);
#5066=VECTOR('',#19028,10.);
#5067=VECTOR('',#19029,10.);
#5068=VECTOR('',#19030,10.);
#5069=VECTOR('',#19031,10.);
#5070=VECTOR('',#19036,10.);
#5071=VECTOR('',#19041,10.);
#5072=VECTOR('',#19042,10.);
#5073=VECTOR('',#19043,10.);
#5074=VECTOR('',#19048,10.);
#5075=VECTOR('',#19053,10.);
#5076=VECTOR('',#19054,10.);
#5077=VECTOR('',#19055,10.);
#5078=VECTOR('',#19060,10.);
#5079=VECTOR('',#19065,10.);
#5080=VECTOR('',#19066,10.);
#5081=VECTOR('',#19067,10.);
#5082=VECTOR('',#19076,10.);
#5083=VECTOR('',#19077,10.);
#5084=VECTOR('',#19078,10.);
#5085=VECTOR('',#19079,10.);
#5086=VECTOR('',#19086,10.);
#5087=VECTOR('',#19089,10.);
#5088=VECTOR('',#19090,10.);
#5089=VECTOR('',#19091,10.);
#5090=VECTOR('',#19098,10.);
#5091=VECTOR('',#19101,10.);
#5092=VECTOR('',#19102,10.);
#5093=VECTOR('',#19103,10.);
#5094=VECTOR('',#19110,10.);
#5095=VECTOR('',#19113,10.);
#5096=VECTOR('',#19114,10.);
#5097=VECTOR('',#19115,10.);
#5709=CIRCLE('',#15819,0.400000000000027);
#5710=CIRCLE('',#15820,0.400000000000027);
#5711=CIRCLE('',#15823,0.399999999999956);
#5712=CIRCLE('',#15824,0.399999999999956);
#5713=CIRCLE('',#15827,0.399999999999945);
#5714=CIRCLE('',#15828,0.399999999999945);
#5715=CIRCLE('',#15831,0.400000000000027);
#5716=CIRCLE('',#15832,0.400000000000027);
#5717=CIRCLE('',#15835,0.399999999999996);
#5718=CIRCLE('',#15836,0.399999999999996);
#5719=CIRCLE('',#15839,0.4);
#5720=CIRCLE('',#15840,0.4);
#5721=CIRCLE('',#15843,0.399999999999996);
#5722=CIRCLE('',#15844,0.399999999999996);
#5723=CIRCLE('',#15847,0.399999999999996);
#5724=CIRCLE('',#15848,0.399999999999996);
#5725=CIRCLE('',#15851,0.600000000000005);
#5726=CIRCLE('',#15852,0.600000000000005);
#5727=CIRCLE('',#15855,0.600000000000005);
#5728=CIRCLE('',#15856,0.600000000000005);
#5729=CIRCLE('',#15859,0.600000000000005);
#5730=CIRCLE('',#15860,0.600000000000005);
#5731=CIRCLE('',#15863,0.600000000000005);
#5732=CIRCLE('',#15864,0.600000000000005);
#5733=CIRCLE('',#15867,0.600000000000005);
#5734=CIRCLE('',#15868,0.600000000000005);
#5735=CIRCLE('',#15871,0.600000000000005);
#5736=CIRCLE('',#15872,0.600000000000005);
#5737=CIRCLE('',#15875,0.600000000000005);
#5738=CIRCLE('',#15876,0.600000000000005);
#5739=CIRCLE('',#15879,0.600000000000005);
#5740=CIRCLE('',#15880,0.600000000000005);
#5741=CIRCLE('',#15883,0.599999999999987);
#5742=CIRCLE('',#15884,0.599999999999987);
#5743=CIRCLE('',#15887,0.599999999999987);
#5744=CIRCLE('',#15888,0.599999999999987);
#5745=CIRCLE('',#15891,0.599999999999987);
#5746=CIRCLE('',#15892,0.599999999999987);
#5747=CIRCLE('',#15895,0.599999999999987);
#5748=CIRCLE('',#15896,0.599999999999987);
#5749=CIRCLE('',#15899,0.599999999999987);
#5750=CIRCLE('',#15900,0.599999999999987);
#5751=CIRCLE('',#15903,0.599999999999987);
#5752=CIRCLE('',#15904,0.599999999999987);
#5753=CIRCLE('',#15907,0.599999999999987);
#5754=CIRCLE('',#15908,0.599999999999987);
#5755=CIRCLE('',#15911,0.599999999999987);
#5756=CIRCLE('',#15912,0.599999999999987);
#5757=CIRCLE('',#15915,0.599999999999987);
#5758=CIRCLE('',#15916,0.599999999999987);
#5759=CIRCLE('',#15919,0.599999999999987);
#5760=CIRCLE('',#15920,0.599999999999987);
#5761=CIRCLE('',#15923,0.599999999999987);
#5762=CIRCLE('',#15924,0.599999999999987);
#5763=CIRCLE('',#15927,0.599999999999987);
#5764=CIRCLE('',#15928,0.599999999999987);
#5765=CIRCLE('',#15931,0.600000000000001);
#5766=CIRCLE('',#15932,0.600000000000001);
#5767=CIRCLE('',#15935,0.600000000000005);
#5768=CIRCLE('',#15936,0.600000000000005);
#5769=CIRCLE('',#15939,0.599999999999998);
#5770=CIRCLE('',#15940,0.599999999999998);
#5771=CIRCLE('',#15943,0.600000000000005);
#5772=CIRCLE('',#15944,0.600000000000005);
#5773=CIRCLE('',#15947,0.600000000000001);
#5774=CIRCLE('',#15948,0.600000000000001);
#5775=CIRCLE('',#15951,0.600000000000005);
#5776=CIRCLE('',#15952,0.600000000000005);
#5777=CIRCLE('',#15955,0.600000000000003);
#5778=CIRCLE('',#15956,0.600000000000003);
#5779=CIRCLE('',#15959,0.600000000000005);
#5780=CIRCLE('',#15960,0.600000000000005);
#5781=CIRCLE('',#15963,0.599999999999996);
#5782=CIRCLE('',#15964,0.599999999999996);
#5783=CIRCLE('',#15967,0.600000000000005);
#5784=CIRCLE('',#15968,0.600000000000005);
#5785=CIRCLE('',#15971,0.599999999999998);
#5786=CIRCLE('',#15972,0.599999999999998);
#5787=CIRCLE('',#15975,0.600000000000005);
#5788=CIRCLE('',#15976,0.600000000000005);
#5789=CIRCLE('',#15979,0.599999999999987);
#5790=CIRCLE('',#15980,0.599999999999987);
#5791=CIRCLE('',#15983,0.599999999999987);
#5792=CIRCLE('',#15984,0.599999999999987);
#5793=CIRCLE('',#15987,0.599999999999987);
#5794=CIRCLE('',#15988,0.599999999999987);
#5795=CIRCLE('',#15991,0.599999999999987);
#5796=CIRCLE('',#15992,0.599999999999987);
#5797=CIRCLE('',#15995,0.600000000000001);
#5798=CIRCLE('',#15996,0.600000000000001);
#5799=CIRCLE('',#15999,0.600000000000005);
#5800=CIRCLE('',#16000,0.600000000000005);
#5801=CIRCLE('',#16003,0.600000000000003);
#5802=CIRCLE('',#16004,0.600000000000003);
#5803=CIRCLE('',#16007,0.600000000000005);
#5804=CIRCLE('',#16008,0.600000000000005);
#5805=CIRCLE('',#16011,0.599999999999987);
#5806=CIRCLE('',#16012,0.599999999999987);
#5807=CIRCLE('',#16015,0.600000000000005);
#5808=CIRCLE('',#16016,0.600000000000005);
#5809=CIRCLE('',#16019,0.600000000000005);
#5810=CIRCLE('',#16020,0.600000000000005);
#5811=CIRCLE('',#16023,0.599999999999987);
#5812=CIRCLE('',#16024,0.599999999999987);
#5813=CIRCLE('',#16027,0.600000000000005);
#5814=CIRCLE('',#16028,0.600000000000005);
#5815=CIRCLE('',#16031,0.600000000000005);
#5816=CIRCLE('',#16032,0.600000000000005);
#5817=CIRCLE('',#16035,0.600000000000005);
#5818=CIRCLE('',#16036,0.600000000000005);
#5819=CIRCLE('',#16039,0.600000000000005);
#5820=CIRCLE('',#16040,0.600000000000005);
#5821=CIRCLE('',#16043,0.600000000000027);
#5822=CIRCLE('',#16044,0.600000000000027);
#5823=CIRCLE('',#16047,0.600000000000023);
#5824=CIRCLE('',#16048,0.600000000000023);
#5825=CIRCLE('',#16051,0.600000000000025);
#5826=CIRCLE('',#16052,0.600000000000025);
#5827=CIRCLE('',#16055,0.600000000000023);
#5828=CIRCLE('',#16056,0.600000000000023);
#5829=CIRCLE('',#16059,1.);
#5830=CIRCLE('',#16060,1.);
#5831=CIRCLE('',#16063,1.00000000000001);
#5832=CIRCLE('',#16064,1.00000000000001);
#5833=CIRCLE('',#16067,1.00000000000001);
#5834=CIRCLE('',#16068,1.00000000000001);
#5835=CIRCLE('',#16071,1.);
#5836=CIRCLE('',#16072,1.);
#6548=VERTEX_POINT('',#22248);
#6549=VERTEX_POINT('',#22249);
#6550=VERTEX_POINT('',#22251);
#6551=VERTEX_POINT('',#22253);
#6552=VERTEX_POINT('',#22257);
#6553=VERTEX_POINT('',#22259);
#6554=VERTEX_POINT('',#22263);
#6555=VERTEX_POINT('',#22265);
#6556=VERTEX_POINT('',#22269);
#6557=VERTEX_POINT('',#22271);
#6558=VERTEX_POINT('',#22275);
#6559=VERTEX_POINT('',#22277);
#6560=VERTEX_POINT('',#22281);
#6561=VERTEX_POINT('',#22283);
#6562=VERTEX_POINT('',#22287);
#6563=VERTEX_POINT('',#22289);
#6564=VERTEX_POINT('',#22296);
#6565=VERTEX_POINT('',#22297);
#6566=VERTEX_POINT('',#22299);
#6567=VERTEX_POINT('',#22301);
#6568=VERTEX_POINT('',#22305);
#6569=VERTEX_POINT('',#22307);
#6570=VERTEX_POINT('',#22311);
#6571=VERTEX_POINT('',#22313);
#6572=VERTEX_POINT('',#22317);
#6573=VERTEX_POINT('',#22319);
#6574=VERTEX_POINT('',#22323);
#6575=VERTEX_POINT('',#22325);
#6576=VERTEX_POINT('',#22329);
#6577=VERTEX_POINT('',#22331);
#6578=VERTEX_POINT('',#22335);
#6579=VERTEX_POINT('',#22337);
#6580=VERTEX_POINT('',#22344);
#6581=VERTEX_POINT('',#22345);
#6582=VERTEX_POINT('',#22347);
#6583=VERTEX_POINT('',#22349);
#6584=VERTEX_POINT('',#22353);
#6585=VERTEX_POINT('',#22355);
#6586=VERTEX_POINT('',#22359);
#6587=VERTEX_POINT('',#22361);
#6588=VERTEX_POINT('',#22365);
#6589=VERTEX_POINT('',#22367);
#6590=VERTEX_POINT('',#22371);
#6591=VERTEX_POINT('',#22373);
#6592=VERTEX_POINT('',#22377);
#6593=VERTEX_POINT('',#22379);
#6594=VERTEX_POINT('',#22383);
#6595=VERTEX_POINT('',#22385);
#6596=VERTEX_POINT('',#22392);
#6597=VERTEX_POINT('',#22393);
#6598=VERTEX_POINT('',#22395);
#6599=VERTEX_POINT('',#22397);
#6600=VERTEX_POINT('',#22401);
#6601=VERTEX_POINT('',#22403);
#6602=VERTEX_POINT('',#22407);
#6603=VERTEX_POINT('',#22409);
#6604=VERTEX_POINT('',#22413);
#6605=VERTEX_POINT('',#22415);
#6606=VERTEX_POINT('',#22419);
#6607=VERTEX_POINT('',#22421);
#6608=VERTEX_POINT('',#22425);
#6609=VERTEX_POINT('',#22427);
#6610=VERTEX_POINT('',#22431);
#6611=VERTEX_POINT('',#22433);
#6612=VERTEX_POINT('',#22440);
#6613=VERTEX_POINT('',#22441);
#6614=VERTEX_POINT('',#22443);
#6615=VERTEX_POINT('',#22445);
#6616=VERTEX_POINT('',#22449);
#6617=VERTEX_POINT('',#22451);
#6618=VERTEX_POINT('',#22455);
#6619=VERTEX_POINT('',#22457);
#6620=VERTEX_POINT('',#22461);
#6621=VERTEX_POINT('',#22463);
#6622=VERTEX_POINT('',#22467);
#6623=VERTEX_POINT('',#22469);
#6624=VERTEX_POINT('',#22473);
#6625=VERTEX_POINT('',#22475);
#6626=VERTEX_POINT('',#22479);
#6627=VERTEX_POINT('',#22481);
#6628=VERTEX_POINT('',#22488);
#6629=VERTEX_POINT('',#22489);
#6630=VERTEX_POINT('',#22491);
#6631=VERTEX_POINT('',#22493);
#6632=VERTEX_POINT('',#22497);
#6633=VERTEX_POINT('',#22499);
#6634=VERTEX_POINT('',#22503);
#6635=VERTEX_POINT('',#22505);
#6636=VERTEX_POINT('',#22509);
#6637=VERTEX_POINT('',#22511);
#6638=VERTEX_POINT('',#22515);
#6639=VERTEX_POINT('',#22517);
#6640=VERTEX_POINT('',#22521);
#6641=VERTEX_POINT('',#22523);
#6642=VERTEX_POINT('',#22527);
#6643=VERTEX_POINT('',#22529);
#6644=VERTEX_POINT('',#22536);
#6645=VERTEX_POINT('',#22537);
#6646=VERTEX_POINT('',#22539);
#6647=VERTEX_POINT('',#22541);
#6648=VERTEX_POINT('',#22545);
#6649=VERTEX_POINT('',#22547);
#6650=VERTEX_POINT('',#22551);
#6651=VERTEX_POINT('',#22553);
#6652=VERTEX_POINT('',#22557);
#6653=VERTEX_POINT('',#22559);
#6654=VERTEX_POINT('',#22563);
#6655=VERTEX_POINT('',#22565);
#6656=VERTEX_POINT('',#22569);
#6657=VERTEX_POINT('',#22571);
#6658=VERTEX_POINT('',#22575);
#6659=VERTEX_POINT('',#22577);
#6660=VERTEX_POINT('',#22584);
#6661=VERTEX_POINT('',#22585);
#6662=VERTEX_POINT('',#22587);
#6663=VERTEX_POINT('',#22589);
#6664=VERTEX_POINT('',#22593);
#6665=VERTEX_POINT('',#22595);
#6666=VERTEX_POINT('',#22599);
#6667=VERTEX_POINT('',#22601);
#6668=VERTEX_POINT('',#22605);
#6669=VERTEX_POINT('',#22607);
#6670=VERTEX_POINT('',#22611);
#6671=VERTEX_POINT('',#22613);
#6672=VERTEX_POINT('',#22617);
#6673=VERTEX_POINT('',#22619);
#6674=VERTEX_POINT('',#22623);
#6675=VERTEX_POINT('',#22625);
#6676=VERTEX_POINT('',#22632);
#6677=VERTEX_POINT('',#22633);
#6678=VERTEX_POINT('',#22635);
#6679=VERTEX_POINT('',#22637);
#6680=VERTEX_POINT('',#22641);
#6681=VERTEX_POINT('',#22643);
#6682=VERTEX_POINT('',#22647);
#6683=VERTEX_POINT('',#22649);
#6684=VERTEX_POINT('',#22653);
#6685=VERTEX_POINT('',#22655);
#6686=VERTEX_POINT('',#22659);
#6687=VERTEX_POINT('',#22661);
#6688=VERTEX_POINT('',#22665);
#6689=VERTEX_POINT('',#22667);
#6690=VERTEX_POINT('',#22671);
#6691=VERTEX_POINT('',#22673);
#6692=VERTEX_POINT('',#22680);
#6693=VERTEX_POINT('',#22681);
#6694=VERTEX_POINT('',#22683);
#6695=VERTEX_POINT('',#22685);
#6696=VERTEX_POINT('',#22689);
#6697=VERTEX_POINT('',#22691);
#6698=VERTEX_POINT('',#22695);
#6699=VERTEX_POINT('',#22697);
#6700=VERTEX_POINT('',#22701);
#6701=VERTEX_POINT('',#22703);
#6702=VERTEX_POINT('',#22707);
#6703=VERTEX_POINT('',#22709);
#6704=VERTEX_POINT('',#22713);
#6705=VERTEX_POINT('',#22715);
#6706=VERTEX_POINT('',#22719);
#6707=VERTEX_POINT('',#22721);
#6708=VERTEX_POINT('',#22728);
#6709=VERTEX_POINT('',#22729);
#6710=VERTEX_POINT('',#22731);
#6711=VERTEX_POINT('',#22733);
#6712=VERTEX_POINT('',#22737);
#6713=VERTEX_POINT('',#22739);
#6714=VERTEX_POINT('',#22743);
#6715=VERTEX_POINT('',#22745);
#6716=VERTEX_POINT('',#22749);
#6717=VERTEX_POINT('',#22751);
#6718=VERTEX_POINT('',#22755);
#6719=VERTEX_POINT('',#22757);
#6720=VERTEX_POINT('',#22761);
#6721=VERTEX_POINT('',#22763);
#6722=VERTEX_POINT('',#22767);
#6723=VERTEX_POINT('',#22769);
#6724=VERTEX_POINT('',#22776);
#6725=VERTEX_POINT('',#22777);
#6726=VERTEX_POINT('',#22779);
#6727=VERTEX_POINT('',#22781);
#6728=VERTEX_POINT('',#22785);
#6729=VERTEX_POINT('',#22787);
#6730=VERTEX_POINT('',#22791);
#6731=VERTEX_POINT('',#22793);
#6732=VERTEX_POINT('',#22797);
#6733=VERTEX_POINT('',#22799);
#6734=VERTEX_POINT('',#22803);
#6735=VERTEX_POINT('',#22805);
#6736=VERTEX_POINT('',#22809);
#6737=VERTEX_POINT('',#22811);
#6738=VERTEX_POINT('',#22815);
#6739=VERTEX_POINT('',#22817);
#6740=VERTEX_POINT('',#22824);
#6741=VERTEX_POINT('',#22825);
#6742=VERTEX_POINT('',#22827);
#6743=VERTEX_POINT('',#22829);
#6744=VERTEX_POINT('',#22833);
#6745=VERTEX_POINT('',#22835);
#6746=VERTEX_POINT('',#22839);
#6747=VERTEX_POINT('',#22841);
#6748=VERTEX_POINT('',#22845);
#6749=VERTEX_POINT('',#22847);
#6750=VERTEX_POINT('',#22851);
#6751=VERTEX_POINT('',#22853);
#6752=VERTEX_POINT('',#22857);
#6753=VERTEX_POINT('',#22859);
#6754=VERTEX_POINT('',#22863);
#6755=VERTEX_POINT('',#22865);
#6756=VERTEX_POINT('',#22872);
#6757=VERTEX_POINT('',#22873);
#6758=VERTEX_POINT('',#22875);
#6759=VERTEX_POINT('',#22877);
#6760=VERTEX_POINT('',#22881);
#6761=VERTEX_POINT('',#22883);
#6762=VERTEX_POINT('',#22887);
#6763=VERTEX_POINT('',#22889);
#6764=VERTEX_POINT('',#22893);
#6765=VERTEX_POINT('',#22895);
#6766=VERTEX_POINT('',#22899);
#6767=VERTEX_POINT('',#22901);
#6768=VERTEX_POINT('',#22905);
#6769=VERTEX_POINT('',#22907);
#6770=VERTEX_POINT('',#22911);
#6771=VERTEX_POINT('',#22913);
#6772=VERTEX_POINT('',#22920);
#6773=VERTEX_POINT('',#22921);
#6774=VERTEX_POINT('',#22923);
#6775=VERTEX_POINT('',#22925);
#6776=VERTEX_POINT('',#22929);
#6777=VERTEX_POINT('',#22931);
#6778=VERTEX_POINT('',#22935);
#6779=VERTEX_POINT('',#22937);
#6780=VERTEX_POINT('',#22941);
#6781=VERTEX_POINT('',#22943);
#6782=VERTEX_POINT('',#22947);
#6783=VERTEX_POINT('',#22949);
#6784=VERTEX_POINT('',#22953);
#6785=VERTEX_POINT('',#22955);
#6786=VERTEX_POINT('',#22959);
#6787=VERTEX_POINT('',#22961);
#6788=VERTEX_POINT('',#22968);
#6789=VERTEX_POINT('',#22969);
#6790=VERTEX_POINT('',#22971);
#6791=VERTEX_POINT('',#22973);
#6792=VERTEX_POINT('',#22977);
#6793=VERTEX_POINT('',#22979);
#6794=VERTEX_POINT('',#22983);
#6795=VERTEX_POINT('',#22985);
#6796=VERTEX_POINT('',#22989);
#6797=VERTEX_POINT('',#22991);
#6798=VERTEX_POINT('',#22995);
#6799=VERTEX_POINT('',#22997);
#6800=VERTEX_POINT('',#23001);
#6801=VERTEX_POINT('',#23003);
#6802=VERTEX_POINT('',#23007);
#6803=VERTEX_POINT('',#23009);
#8363=EDGE_CURVE('',#6548,#6549,#3730,.T.);
#8364=EDGE_CURVE('',#6548,#6550,#3731,.T.);
#8365=EDGE_CURVE('',#6551,#6550,#3732,.T.);
#8366=EDGE_CURVE('',#6549,#6551,#3733,.T.);
#8367=EDGE_CURVE('',#6552,#6548,#5709,.T.);
#8368=EDGE_CURVE('',#6552,#6553,#3734,.T.);
#8369=EDGE_CURVE('',#6550,#6553,#5710,.T.);
#8370=EDGE_CURVE('',#6554,#6552,#3735,.T.);
#8371=EDGE_CURVE('',#6554,#6555,#3736,.T.);
#8372=EDGE_CURVE('',#6553,#6555,#3737,.T.);
#8373=EDGE_CURVE('',#6556,#6554,#5711,.T.);
#8374=EDGE_CURVE('',#6556,#6557,#3738,.T.);
#8375=EDGE_CURVE('',#6555,#6557,#5712,.T.);
#8376=EDGE_CURVE('',#6558,#6556,#3739,.T.);
#8377=EDGE_CURVE('',#6558,#6559,#3740,.T.);
#8378=EDGE_CURVE('',#6557,#6559,#3741,.T.);
#8379=EDGE_CURVE('',#6560,#6558,#5713,.T.);
#8380=EDGE_CURVE('',#6560,#6561,#3742,.T.);
#8381=EDGE_CURVE('',#6559,#6561,#5714,.T.);
#8382=EDGE_CURVE('',#6562,#6560,#3743,.T.);
#8383=EDGE_CURVE('',#6562,#6563,#3744,.T.);
#8384=EDGE_CURVE('',#6561,#6563,#3745,.T.);
#8385=EDGE_CURVE('',#6549,#6562,#5715,.T.);
#8386=EDGE_CURVE('',#6563,#6551,#5716,.T.);
#8387=EDGE_CURVE('',#6564,#6565,#3746,.T.);
#8388=EDGE_CURVE('',#6564,#6566,#3747,.T.);
#8389=EDGE_CURVE('',#6567,#6566,#3748,.T.);
#8390=EDGE_CURVE('',#6565,#6567,#3749,.T.);
#8391=EDGE_CURVE('',#6568,#6564,#5717,.T.);
#8392=EDGE_CURVE('',#6568,#6569,#3750,.T.);
#8393=EDGE_CURVE('',#6566,#6569,#5718,.T.);
#8394=EDGE_CURVE('',#6570,#6568,#3751,.T.);
#8395=EDGE_CURVE('',#6570,#6571,#3752,.T.);
#8396=EDGE_CURVE('',#6569,#6571,#3753,.T.);
#8397=EDGE_CURVE('',#6572,#6570,#5719,.T.);
#8398=EDGE_CURVE('',#6572,#6573,#3754,.T.);
#8399=EDGE_CURVE('',#6571,#6573,#5720,.T.);
#8400=EDGE_CURVE('',#6574,#6572,#3755,.T.);
#8401=EDGE_CURVE('',#6574,#6575,#3756,.T.);
#8402=EDGE_CURVE('',#6573,#6575,#3757,.T.);
#8403=EDGE_CURVE('',#6576,#6574,#5721,.T.);
#8404=EDGE_CURVE('',#6576,#6577,#3758,.T.);
#8405=EDGE_CURVE('',#6575,#6577,#5722,.T.);
#8406=EDGE_CURVE('',#6578,#6576,#3759,.T.);
#8407=EDGE_CURVE('',#6578,#6579,#3760,.T.);
#8408=EDGE_CURVE('',#6577,#6579,#3761,.T.);
#8409=EDGE_CURVE('',#6565,#6578,#5723,.T.);
#8410=EDGE_CURVE('',#6579,#6567,#5724,.T.);
#8411=EDGE_CURVE('',#6580,#6581,#3762,.T.);
#8412=EDGE_CURVE('',#6580,#6582,#3763,.T.);
#8413=EDGE_CURVE('',#6583,#6582,#3764,.T.);
#8414=EDGE_CURVE('',#6581,#6583,#3765,.T.);
#8415=EDGE_CURVE('',#6584,#6580,#5725,.T.);
#8416=EDGE_CURVE('',#6584,#6585,#3766,.T.);
#8417=EDGE_CURVE('',#6582,#6585,#5726,.T.);
#8418=EDGE_CURVE('',#6586,#6584,#3767,.T.);
#8419=EDGE_CURVE('',#6586,#6587,#3768,.T.);
#8420=EDGE_CURVE('',#6585,#6587,#3769,.T.);
#8421=EDGE_CURVE('',#6588,#6586,#5727,.T.);
#8422=EDGE_CURVE('',#6588,#6589,#3770,.T.);
#8423=EDGE_CURVE('',#6587,#6589,#5728,.T.);
#8424=EDGE_CURVE('',#6590,#6588,#3771,.T.);
#8425=EDGE_CURVE('',#6590,#6591,#3772,.T.);
#8426=EDGE_CURVE('',#6589,#6591,#3773,.T.);
#8427=EDGE_CURVE('',#6592,#6590,#5729,.T.);
#8428=EDGE_CURVE('',#6592,#6593,#3774,.T.);
#8429=EDGE_CURVE('',#6591,#6593,#5730,.T.);
#8430=EDGE_CURVE('',#6594,#6592,#3775,.T.);
#8431=EDGE_CURVE('',#6594,#6595,#3776,.T.);
#8432=EDGE_CURVE('',#6593,#6595,#3777,.T.);
#8433=EDGE_CURVE('',#6581,#6594,#5731,.T.);
#8434=EDGE_CURVE('',#6595,#6583,#5732,.T.);
#8435=EDGE_CURVE('',#6596,#6597,#3778,.T.);
#8436=EDGE_CURVE('',#6596,#6598,#3779,.T.);
#8437=EDGE_CURVE('',#6599,#6598,#3780,.T.);
#8438=EDGE_CURVE('',#6597,#6599,#3781,.T.);
#8439=EDGE_CURVE('',#6600,#6596,#5733,.T.);
#8440=EDGE_CURVE('',#6600,#6601,#3782,.T.);
#8441=EDGE_CURVE('',#6598,#6601,#5734,.T.);
#8442=EDGE_CURVE('',#6602,#6600,#3783,.T.);
#8443=EDGE_CURVE('',#6602,#6603,#3784,.T.);
#8444=EDGE_CURVE('',#6601,#6603,#3785,.T.);
#8445=EDGE_CURVE('',#6604,#6602,#5735,.T.);
#8446=EDGE_CURVE('',#6604,#6605,#3786,.T.);
#8447=EDGE_CURVE('',#6603,#6605,#5736,.T.);
#8448=EDGE_CURVE('',#6606,#6604,#3787,.T.);
#8449=EDGE_CURVE('',#6606,#6607,#3788,.T.);
#8450=EDGE_CURVE('',#6605,#6607,#3789,.T.);
#8451=EDGE_CURVE('',#6608,#6606,#5737,.T.);
#8452=EDGE_CURVE('',#6608,#6609,#3790,.T.);
#8453=EDGE_CURVE('',#6607,#6609,#5738,.T.);
#8454=EDGE_CURVE('',#6610,#6608,#3791,.T.);
#8455=EDGE_CURVE('',#6610,#6611,#3792,.T.);
#8456=EDGE_CURVE('',#6609,#6611,#3793,.T.);
#8457=EDGE_CURVE('',#6597,#6610,#5739,.T.);
#8458=EDGE_CURVE('',#6611,#6599,#5740,.T.);
#8459=EDGE_CURVE('',#6612,#6613,#3794,.T.);
#8460=EDGE_CURVE('',#6612,#6614,#3795,.T.);
#8461=EDGE_CURVE('',#6615,#6614,#3796,.T.);
#8462=EDGE_CURVE('',#6613,#6615,#3797,.T.);
#8463=EDGE_CURVE('',#6616,#6612,#5741,.T.);
#8464=EDGE_CURVE('',#6616,#6617,#3798,.T.);
#8465=EDGE_CURVE('',#6614,#6617,#5742,.T.);
#8466=EDGE_CURVE('',#6618,#6616,#3799,.T.);
#8467=EDGE_CURVE('',#6618,#6619,#3800,.T.);
#8468=EDGE_CURVE('',#6617,#6619,#3801,.T.);
#8469=EDGE_CURVE('',#6620,#6618,#5743,.T.);
#8470=EDGE_CURVE('',#6620,#6621,#3802,.T.);
#8471=EDGE_CURVE('',#6619,#6621,#5744,.T.);
#8472=EDGE_CURVE('',#6622,#6620,#3803,.T.);
#8473=EDGE_CURVE('',#6622,#6623,#3804,.T.);
#8474=EDGE_CURVE('',#6621,#6623,#3805,.T.);
#8475=EDGE_CURVE('',#6624,#6622,#5745,.T.);
#8476=EDGE_CURVE('',#6624,#6625,#3806,.T.);
#8477=EDGE_CURVE('',#6623,#6625,#5746,.T.);
#8478=EDGE_CURVE('',#6626,#6624,#3807,.T.);
#8479=EDGE_CURVE('',#6626,#6627,#3808,.T.);
#8480=EDGE_CURVE('',#6625,#6627,#3809,.T.);
#8481=EDGE_CURVE('',#6613,#6626,#5747,.T.);
#8482=EDGE_CURVE('',#6627,#6615,#5748,.T.);
#8483=EDGE_CURVE('',#6628,#6629,#3810,.T.);
#8484=EDGE_CURVE('',#6628,#6630,#3811,.T.);
#8485=EDGE_CURVE('',#6631,#6630,#3812,.T.);
#8486=EDGE_CURVE('',#6629,#6631,#3813,.T.);
#8487=EDGE_CURVE('',#6632,#6628,#5749,.T.);
#8488=EDGE_CURVE('',#6632,#6633,#3814,.T.);
#8489=EDGE_CURVE('',#6630,#6633,#5750,.T.);
#8490=EDGE_CURVE('',#6634,#6632,#3815,.T.);
#8491=EDGE_CURVE('',#6634,#6635,#3816,.T.);
#8492=EDGE_CURVE('',#6633,#6635,#3817,.T.);
#8493=EDGE_CURVE('',#6636,#6634,#5751,.T.);
#8494=EDGE_CURVE('',#6636,#6637,#3818,.T.);
#8495=EDGE_CURVE('',#6635,#6637,#5752,.T.);
#8496=EDGE_CURVE('',#6638,#6636,#3819,.T.);
#8497=EDGE_CURVE('',#6638,#6639,#3820,.T.);
#8498=EDGE_CURVE('',#6637,#6639,#3821,.T.);
#8499=EDGE_CURVE('',#6640,#6638,#5753,.T.);
#8500=EDGE_CURVE('',#6640,#6641,#3822,.T.);
#8501=EDGE_CURVE('',#6639,#6641,#5754,.T.);
#8502=EDGE_CURVE('',#6642,#6640,#3823,.T.);
#8503=EDGE_CURVE('',#6642,#6643,#3824,.T.);
#8504=EDGE_CURVE('',#6641,#6643,#3825,.T.);
#8505=EDGE_CURVE('',#6629,#6642,#5755,.T.);
#8506=EDGE_CURVE('',#6643,#6631,#5756,.T.);
#8507=EDGE_CURVE('',#6644,#6645,#3826,.T.);
#8508=EDGE_CURVE('',#6644,#6646,#3827,.T.);
#8509=EDGE_CURVE('',#6647,#6646,#3828,.T.);
#8510=EDGE_CURVE('',#6645,#6647,#3829,.T.);
#8511=EDGE_CURVE('',#6648,#6644,#5757,.T.);
#8512=EDGE_CURVE('',#6648,#6649,#3830,.T.);
#8513=EDGE_CURVE('',#6646,#6649,#5758,.T.);
#8514=EDGE_CURVE('',#6650,#6648,#3831,.T.);
#8515=EDGE_CURVE('',#6650,#6651,#3832,.T.);
#8516=EDGE_CURVE('',#6649,#6651,#3833,.T.);
#8517=EDGE_CURVE('',#6652,#6650,#5759,.T.);
#8518=EDGE_CURVE('',#6652,#6653,#3834,.T.);
#8519=EDGE_CURVE('',#6651,#6653,#5760,.T.);
#8520=EDGE_CURVE('',#6654,#6652,#3835,.T.);
#8521=EDGE_CURVE('',#6654,#6655,#3836,.T.);
#8522=EDGE_CURVE('',#6653,#6655,#3837,.T.);
#8523=EDGE_CURVE('',#6656,#6654,#5761,.T.);
#8524=EDGE_CURVE('',#6656,#6657,#3838,.T.);
#8525=EDGE_CURVE('',#6655,#6657,#5762,.T.);
#8526=EDGE_CURVE('',#6658,#6656,#3839,.T.);
#8527=EDGE_CURVE('',#6658,#6659,#3840,.T.);
#8528=EDGE_CURVE('',#6657,#6659,#3841,.T.);
#8529=EDGE_CURVE('',#6645,#6658,#5763,.T.);
#8530=EDGE_CURVE('',#6659,#6647,#5764,.T.);
#8531=EDGE_CURVE('',#6660,#6661,#3842,.T.);
#8532=EDGE_CURVE('',#6660,#6662,#3843,.T.);
#8533=EDGE_CURVE('',#6663,#6662,#3844,.T.);
#8534=EDGE_CURVE('',#6661,#6663,#3845,.T.);
#8535=EDGE_CURVE('',#6664,#6660,#5765,.T.);
#8536=EDGE_CURVE('',#6664,#6665,#3846,.T.);
#8537=EDGE_CURVE('',#6662,#6665,#5766,.T.);
#8538=EDGE_CURVE('',#6666,#6664,#3847,.T.);
#8539=EDGE_CURVE('',#6666,#6667,#3848,.T.);
#8540=EDGE_CURVE('',#6665,#6667,#3849,.T.);
#8541=EDGE_CURVE('',#6668,#6666,#5767,.T.);
#8542=EDGE_CURVE('',#6668,#6669,#3850,.T.);
#8543=EDGE_CURVE('',#6667,#6669,#5768,.T.);
#8544=EDGE_CURVE('',#6670,#6668,#3851,.T.);
#8545=EDGE_CURVE('',#6670,#6671,#3852,.T.);
#8546=EDGE_CURVE('',#6669,#6671,#3853,.T.);
#8547=EDGE_CURVE('',#6672,#6670,#5769,.T.);
#8548=EDGE_CURVE('',#6672,#6673,#3854,.T.);
#8549=EDGE_CURVE('',#6671,#6673,#5770,.T.);
#8550=EDGE_CURVE('',#6674,#6672,#3855,.T.);
#8551=EDGE_CURVE('',#6674,#6675,#3856,.T.);
#8552=EDGE_CURVE('',#6673,#6675,#3857,.T.);
#8553=EDGE_CURVE('',#6661,#6674,#5771,.T.);
#8554=EDGE_CURVE('',#6675,#6663,#5772,.T.);
#8555=EDGE_CURVE('',#6676,#6677,#3858,.T.);
#8556=EDGE_CURVE('',#6676,#6678,#3859,.T.);
#8557=EDGE_CURVE('',#6679,#6678,#3860,.T.);
#8558=EDGE_CURVE('',#6677,#6679,#3861,.T.);
#8559=EDGE_CURVE('',#6680,#6676,#5773,.T.);
#8560=EDGE_CURVE('',#6680,#6681,#3862,.T.);
#8561=EDGE_CURVE('',#6678,#6681,#5774,.T.);
#8562=EDGE_CURVE('',#6682,#6680,#3863,.T.);
#8563=EDGE_CURVE('',#6682,#6683,#3864,.T.);
#8564=EDGE_CURVE('',#6681,#6683,#3865,.T.);
#8565=EDGE_CURVE('',#6684,#6682,#5775,.T.);
#8566=EDGE_CURVE('',#6684,#6685,#3866,.T.);
#8567=EDGE_CURVE('',#6683,#6685,#5776,.T.);
#8568=EDGE_CURVE('',#6686,#6684,#3867,.T.);
#8569=EDGE_CURVE('',#6686,#6687,#3868,.T.);
#8570=EDGE_CURVE('',#6685,#6687,#3869,.T.);
#8571=EDGE_CURVE('',#6688,#6686,#5777,.T.);
#8572=EDGE_CURVE('',#6688,#6689,#3870,.T.);
#8573=EDGE_CURVE('',#6687,#6689,#5778,.T.);
#8574=EDGE_CURVE('',#6690,#6688,#3871,.T.);
#8575=EDGE_CURVE('',#6690,#6691,#3872,.T.);
#8576=EDGE_CURVE('',#6689,#6691,#3873,.T.);
#8577=EDGE_CURVE('',#6677,#6690,#5779,.T.);
#8578=EDGE_CURVE('',#6691,#6679,#5780,.T.);
#8579=EDGE_CURVE('',#6692,#6693,#3874,.T.);
#8580=EDGE_CURVE('',#6692,#6694,#3875,.T.);
#8581=EDGE_CURVE('',#6695,#6694,#3876,.T.);
#8582=EDGE_CURVE('',#6693,#6695,#3877,.T.);
#8583=EDGE_CURVE('',#6696,#6692,#5781,.T.);
#8584=EDGE_CURVE('',#6696,#6697,#3878,.T.);
#8585=EDGE_CURVE('',#6694,#6697,#5782,.T.);
#8586=EDGE_CURVE('',#6698,#6696,#3879,.T.);
#8587=EDGE_CURVE('',#6698,#6699,#3880,.T.);
#8588=EDGE_CURVE('',#6697,#6699,#3881,.T.);
#8589=EDGE_CURVE('',#6700,#6698,#5783,.T.);
#8590=EDGE_CURVE('',#6700,#6701,#3882,.T.);
#8591=EDGE_CURVE('',#6699,#6701,#5784,.T.);
#8592=EDGE_CURVE('',#6702,#6700,#3883,.T.);
#8593=EDGE_CURVE('',#6702,#6703,#3884,.T.);
#8594=EDGE_CURVE('',#6701,#6703,#3885,.T.);
#8595=EDGE_CURVE('',#6704,#6702,#5785,.T.);
#8596=EDGE_CURVE('',#6704,#6705,#3886,.T.);
#8597=EDGE_CURVE('',#6703,#6705,#5786,.T.);
#8598=EDGE_CURVE('',#6706,#6704,#3887,.T.);
#8599=EDGE_CURVE('',#6706,#6707,#3888,.T.);
#8600=EDGE_CURVE('',#6705,#6707,#3889,.T.);
#8601=EDGE_CURVE('',#6693,#6706,#5787,.T.);
#8602=EDGE_CURVE('',#6707,#6695,#5788,.T.);
#8603=EDGE_CURVE('',#6708,#6709,#3890,.T.);
#8604=EDGE_CURVE('',#6708,#6710,#3891,.T.);
#8605=EDGE_CURVE('',#6711,#6710,#3892,.T.);
#8606=EDGE_CURVE('',#6709,#6711,#3893,.T.);
#8607=EDGE_CURVE('',#6712,#6708,#5789,.T.);
#8608=EDGE_CURVE('',#6712,#6713,#3894,.T.);
#8609=EDGE_CURVE('',#6710,#6713,#5790,.T.);
#8610=EDGE_CURVE('',#6714,#6712,#3895,.T.);
#8611=EDGE_CURVE('',#6714,#6715,#3896,.T.);
#8612=EDGE_CURVE('',#6713,#6715,#3897,.T.);
#8613=EDGE_CURVE('',#6716,#6714,#5791,.T.);
#8614=EDGE_CURVE('',#6716,#6717,#3898,.T.);
#8615=EDGE_CURVE('',#6715,#6717,#5792,.T.);
#8616=EDGE_CURVE('',#6718,#6716,#3899,.T.);
#8617=EDGE_CURVE('',#6718,#6719,#3900,.T.);
#8618=EDGE_CURVE('',#6717,#6719,#3901,.T.);
#8619=EDGE_CURVE('',#6720,#6718,#5793,.T.);
#8620=EDGE_CURVE('',#6720,#6721,#3902,.T.);
#8621=EDGE_CURVE('',#6719,#6721,#5794,.T.);
#8622=EDGE_CURVE('',#6722,#6720,#3903,.T.);
#8623=EDGE_CURVE('',#6722,#6723,#3904,.T.);
#8624=EDGE_CURVE('',#6721,#6723,#3905,.T.);
#8625=EDGE_CURVE('',#6709,#6722,#5795,.T.);
#8626=EDGE_CURVE('',#6723,#6711,#5796,.T.);
#8627=EDGE_CURVE('',#6724,#6725,#3906,.T.);
#8628=EDGE_CURVE('',#6724,#6726,#3907,.T.);
#8629=EDGE_CURVE('',#6727,#6726,#3908,.T.);
#8630=EDGE_CURVE('',#6725,#6727,#3909,.T.);
#8631=EDGE_CURVE('',#6728,#6724,#5797,.T.);
#8632=EDGE_CURVE('',#6728,#6729,#3910,.T.);
#8633=EDGE_CURVE('',#6726,#6729,#5798,.T.);
#8634=EDGE_CURVE('',#6730,#6728,#3911,.T.);
#8635=EDGE_CURVE('',#6730,#6731,#3912,.T.);
#8636=EDGE_CURVE('',#6729,#6731,#3913,.T.);
#8637=EDGE_CURVE('',#6732,#6730,#5799,.T.);
#8638=EDGE_CURVE('',#6732,#6733,#3914,.T.);
#8639=EDGE_CURVE('',#6731,#6733,#5800,.T.);
#8640=EDGE_CURVE('',#6734,#6732,#3915,.T.);
#8641=EDGE_CURVE('',#6734,#6735,#3916,.T.);
#8642=EDGE_CURVE('',#6733,#6735,#3917,.T.);
#8643=EDGE_CURVE('',#6736,#6734,#5801,.T.);
#8644=EDGE_CURVE('',#6736,#6737,#3918,.T.);
#8645=EDGE_CURVE('',#6735,#6737,#5802,.T.);
#8646=EDGE_CURVE('',#6738,#6736,#3919,.T.);
#8647=EDGE_CURVE('',#6738,#6739,#3920,.T.);
#8648=EDGE_CURVE('',#6737,#6739,#3921,.T.);
#8649=EDGE_CURVE('',#6725,#6738,#5803,.T.);
#8650=EDGE_CURVE('',#6739,#6727,#5804,.T.);
#8651=EDGE_CURVE('',#6740,#6741,#3922,.T.);
#8652=EDGE_CURVE('',#6740,#6742,#3923,.T.);
#8653=EDGE_CURVE('',#6743,#6742,#3924,.T.);
#8654=EDGE_CURVE('',#6741,#6743,#3925,.T.);
#8655=EDGE_CURVE('',#6744,#6740,#5805,.T.);
#8656=EDGE_CURVE('',#6744,#6745,#3926,.T.);
#8657=EDGE_CURVE('',#6742,#6745,#5806,.T.);
#8658=EDGE_CURVE('',#6746,#6744,#3927,.T.);
#8659=EDGE_CURVE('',#6746,#6747,#3928,.T.);
#8660=EDGE_CURVE('',#6745,#6747,#3929,.T.);
#8661=EDGE_CURVE('',#6748,#6746,#5807,.T.);
#8662=EDGE_CURVE('',#6748,#6749,#3930,.T.);
#8663=EDGE_CURVE('',#6747,#6749,#5808,.T.);
#8664=EDGE_CURVE('',#6750,#6748,#3931,.T.);
#8665=EDGE_CURVE('',#6750,#6751,#3932,.T.);
#8666=EDGE_CURVE('',#6749,#6751,#3933,.T.);
#8667=EDGE_CURVE('',#6752,#6750,#5809,.T.);
#8668=EDGE_CURVE('',#6752,#6753,#3934,.T.);
#8669=EDGE_CURVE('',#6751,#6753,#5810,.T.);
#8670=EDGE_CURVE('',#6754,#6752,#3935,.T.);
#8671=EDGE_CURVE('',#6754,#6755,#3936,.T.);
#8672=EDGE_CURVE('',#6753,#6755,#3937,.T.);
#8673=EDGE_CURVE('',#6741,#6754,#5811,.T.);
#8674=EDGE_CURVE('',#6755,#6743,#5812,.T.);
#8675=EDGE_CURVE('',#6756,#6757,#3938,.T.);
#8676=EDGE_CURVE('',#6756,#6758,#3939,.T.);
#8677=EDGE_CURVE('',#6759,#6758,#3940,.T.);
#8678=EDGE_CURVE('',#6757,#6759,#3941,.T.);
#8679=EDGE_CURVE('',#6760,#6756,#5813,.T.);
#8680=EDGE_CURVE('',#6760,#6761,#3942,.T.);
#8681=EDGE_CURVE('',#6758,#6761,#5814,.T.);
#8682=EDGE_CURVE('',#6762,#6760,#3943,.T.);
#8683=EDGE_CURVE('',#6762,#6763,#3944,.T.);
#8684=EDGE_CURVE('',#6761,#6763,#3945,.T.);
#8685=EDGE_CURVE('',#6764,#6762,#5815,.T.);
#8686=EDGE_CURVE('',#6764,#6765,#3946,.T.);
#8687=EDGE_CURVE('',#6763,#6765,#5816,.T.);
#8688=EDGE_CURVE('',#6766,#6764,#3947,.T.);
#8689=EDGE_CURVE('',#6766,#6767,#3948,.T.);
#8690=EDGE_CURVE('',#6765,#6767,#3949,.T.);
#8691=EDGE_CURVE('',#6768,#6766,#5817,.T.);
#8692=EDGE_CURVE('',#6768,#6769,#3950,.T.);
#8693=EDGE_CURVE('',#6767,#6769,#5818,.T.);
#8694=EDGE_CURVE('',#6770,#6768,#3951,.T.);
#8695=EDGE_CURVE('',#6770,#6771,#3952,.T.);
#8696=EDGE_CURVE('',#6769,#6771,#3953,.T.);
#8697=EDGE_CURVE('',#6757,#6770,#5819,.T.);
#8698=EDGE_CURVE('',#6771,#6759,#5820,.T.);
#8699=EDGE_CURVE('',#6772,#6773,#3954,.T.);
#8700=EDGE_CURVE('',#6772,#6774,#3955,.T.);
#8701=EDGE_CURVE('',#6775,#6774,#3956,.T.);
#8702=EDGE_CURVE('',#6773,#6775,#3957,.T.);
#8703=EDGE_CURVE('',#6776,#6772,#5821,.T.);
#8704=EDGE_CURVE('',#6776,#6777,#3958,.T.);
#8705=EDGE_CURVE('',#6774,#6777,#5822,.T.);
#8706=EDGE_CURVE('',#6778,#6776,#3959,.T.);
#8707=EDGE_CURVE('',#6778,#6779,#3960,.T.);
#8708=EDGE_CURVE('',#6777,#6779,#3961,.T.);
#8709=EDGE_CURVE('',#6780,#6778,#5823,.T.);
#8710=EDGE_CURVE('',#6780,#6781,#3962,.T.);
#8711=EDGE_CURVE('',#6779,#6781,#5824,.T.);
#8712=EDGE_CURVE('',#6782,#6780,#3963,.T.);
#8713=EDGE_CURVE('',#6782,#6783,#3964,.T.);
#8714=EDGE_CURVE('',#6781,#6783,#3965,.T.);
#8715=EDGE_CURVE('',#6784,#6782,#5825,.T.);
#8716=EDGE_CURVE('',#6784,#6785,#3966,.T.);
#8717=EDGE_CURVE('',#6783,#6785,#5826,.T.);
#8718=EDGE_CURVE('',#6786,#6784,#3967,.T.);
#8719=EDGE_CURVE('',#6786,#6787,#3968,.T.);
#8720=EDGE_CURVE('',#6785,#6787,#3969,.T.);
#8721=EDGE_CURVE('',#6773,#6786,#5827,.T.);
#8722=EDGE_CURVE('',#6787,#6775,#5828,.T.);
#8723=EDGE_CURVE('',#6788,#6789,#3970,.T.);
#8724=EDGE_CURVE('',#6789,#6790,#3971,.T.);
#8725=EDGE_CURVE('',#6791,#6790,#3972,.T.);
#8726=EDGE_CURVE('',#6788,#6791,#3973,.T.);
#8727=EDGE_CURVE('',#6792,#6788,#5829,.T.);
#8728=EDGE_CURVE('',#6793,#6791,#5830,.T.);
#8729=EDGE_CURVE('',#6792,#6793,#3974,.T.);
#8730=EDGE_CURVE('',#6794,#6792,#3975,.T.);
#8731=EDGE_CURVE('',#6795,#6793,#3976,.T.);
#8732=EDGE_CURVE('',#6794,#6795,#3977,.T.);
#8733=EDGE_CURVE('',#6796,#6794,#5831,.T.);
#8734=EDGE_CURVE('',#6797,#6795,#5832,.T.);
#8735=EDGE_CURVE('',#6796,#6797,#3978,.T.);
#8736=EDGE_CURVE('',#6798,#6796,#3979,.T.);
#8737=EDGE_CURVE('',#6799,#6797,#3980,.T.);
#8738=EDGE_CURVE('',#6798,#6799,#3981,.T.);
#8739=EDGE_CURVE('',#6800,#6798,#5833,.T.);
#8740=EDGE_CURVE('',#6801,#6799,#5834,.T.);
#8741=EDGE_CURVE('',#6800,#6801,#3982,.T.);
#8742=EDGE_CURVE('',#6802,#6800,#3983,.T.);
#8743=EDGE_CURVE('',#6803,#6801,#3984,.T.);
#8744=EDGE_CURVE('',#6802,#6803,#3985,.T.);
#8745=EDGE_CURVE('',#6789,#6802,#5835,.T.);
#8746=EDGE_CURVE('',#6790,#6803,#5836,.T.);
#11400=ORIENTED_EDGE('',*,*,#8363,.F.);
#11401=ORIENTED_EDGE('',*,*,#8364,.T.);
#11402=ORIENTED_EDGE('',*,*,#8365,.F.);
#11403=ORIENTED_EDGE('',*,*,#8366,.F.);
#11404=ORIENTED_EDGE('',*,*,#8367,.F.);
#11405=ORIENTED_EDGE('',*,*,#8368,.T.);
#11406=ORIENTED_EDGE('',*,*,#8369,.F.);
#11407=ORIENTED_EDGE('',*,*,#8364,.F.);
#11408=ORIENTED_EDGE('',*,*,#8370,.F.);
#11409=ORIENTED_EDGE('',*,*,#8371,.T.);
#11410=ORIENTED_EDGE('',*,*,#8372,.F.);
#11411=ORIENTED_EDGE('',*,*,#8368,.F.);
#11412=ORIENTED_EDGE('',*,*,#8373,.F.);
#11413=ORIENTED_EDGE('',*,*,#8374,.T.);
#11414=ORIENTED_EDGE('',*,*,#8375,.F.);
#11415=ORIENTED_EDGE('',*,*,#8371,.F.);
#11416=ORIENTED_EDGE('',*,*,#8376,.F.);
#11417=ORIENTED_EDGE('',*,*,#8377,.T.);
#11418=ORIENTED_EDGE('',*,*,#8378,.F.);
#11419=ORIENTED_EDGE('',*,*,#8374,.F.);
#11420=ORIENTED_EDGE('',*,*,#8379,.F.);
#11421=ORIENTED_EDGE('',*,*,#8380,.T.);
#11422=ORIENTED_EDGE('',*,*,#8381,.F.);
#11423=ORIENTED_EDGE('',*,*,#8377,.F.);
#11424=ORIENTED_EDGE('',*,*,#8382,.F.);
#11425=ORIENTED_EDGE('',*,*,#8383,.T.);
#11426=ORIENTED_EDGE('',*,*,#8384,.F.);
#11427=ORIENTED_EDGE('',*,*,#8380,.F.);
#11428=ORIENTED_EDGE('',*,*,#8385,.F.);
#11429=ORIENTED_EDGE('',*,*,#8366,.T.);
#11430=ORIENTED_EDGE('',*,*,#8386,.F.);
#11431=ORIENTED_EDGE('',*,*,#8383,.F.);
#11432=ORIENTED_EDGE('',*,*,#8387,.F.);
#11433=ORIENTED_EDGE('',*,*,#8388,.T.);
#11434=ORIENTED_EDGE('',*,*,#8389,.F.);
#11435=ORIENTED_EDGE('',*,*,#8390,.F.);
#11436=ORIENTED_EDGE('',*,*,#8391,.F.);
#11437=ORIENTED_EDGE('',*,*,#8392,.T.);
#11438=ORIENTED_EDGE('',*,*,#8393,.F.);
#11439=ORIENTED_EDGE('',*,*,#8388,.F.);
#11440=ORIENTED_EDGE('',*,*,#8394,.F.);
#11441=ORIENTED_EDGE('',*,*,#8395,.T.);
#11442=ORIENTED_EDGE('',*,*,#8396,.F.);
#11443=ORIENTED_EDGE('',*,*,#8392,.F.);
#11444=ORIENTED_EDGE('',*,*,#8397,.F.);
#11445=ORIENTED_EDGE('',*,*,#8398,.T.);
#11446=ORIENTED_EDGE('',*,*,#8399,.F.);
#11447=ORIENTED_EDGE('',*,*,#8395,.F.);
#11448=ORIENTED_EDGE('',*,*,#8400,.F.);
#11449=ORIENTED_EDGE('',*,*,#8401,.T.);
#11450=ORIENTED_EDGE('',*,*,#8402,.F.);
#11451=ORIENTED_EDGE('',*,*,#8398,.F.);
#11452=ORIENTED_EDGE('',*,*,#8403,.F.);
#11453=ORIENTED_EDGE('',*,*,#8404,.T.);
#11454=ORIENTED_EDGE('',*,*,#8405,.F.);
#11455=ORIENTED_EDGE('',*,*,#8401,.F.);
#11456=ORIENTED_EDGE('',*,*,#8406,.F.);
#11457=ORIENTED_EDGE('',*,*,#8407,.T.);
#11458=ORIENTED_EDGE('',*,*,#8408,.F.);
#11459=ORIENTED_EDGE('',*,*,#8404,.F.);
#11460=ORIENTED_EDGE('',*,*,#8409,.F.);
#11461=ORIENTED_EDGE('',*,*,#8390,.T.);
#11462=ORIENTED_EDGE('',*,*,#8410,.F.);
#11463=ORIENTED_EDGE('',*,*,#8407,.F.);
#11464=ORIENTED_EDGE('',*,*,#8411,.F.);
#11465=ORIENTED_EDGE('',*,*,#8412,.T.);
#11466=ORIENTED_EDGE('',*,*,#8413,.F.);
#11467=ORIENTED_EDGE('',*,*,#8414,.F.);
#11468=ORIENTED_EDGE('',*,*,#8415,.F.);
#11469=ORIENTED_EDGE('',*,*,#8416,.T.);
#11470=ORIENTED_EDGE('',*,*,#8417,.F.);
#11471=ORIENTED_EDGE('',*,*,#8412,.F.);
#11472=ORIENTED_EDGE('',*,*,#8418,.F.);
#11473=ORIENTED_EDGE('',*,*,#8419,.T.);
#11474=ORIENTED_EDGE('',*,*,#8420,.F.);
#11475=ORIENTED_EDGE('',*,*,#8416,.F.);
#11476=ORIENTED_EDGE('',*,*,#8421,.F.);
#11477=ORIENTED_EDGE('',*,*,#8422,.T.);
#11478=ORIENTED_EDGE('',*,*,#8423,.F.);
#11479=ORIENTED_EDGE('',*,*,#8419,.F.);
#11480=ORIENTED_EDGE('',*,*,#8424,.F.);
#11481=ORIENTED_EDGE('',*,*,#8425,.T.);
#11482=ORIENTED_EDGE('',*,*,#8426,.F.);
#11483=ORIENTED_EDGE('',*,*,#8422,.F.);
#11484=ORIENTED_EDGE('',*,*,#8427,.F.);
#11485=ORIENTED_EDGE('',*,*,#8428,.T.);
#11486=ORIENTED_EDGE('',*,*,#8429,.F.);
#11487=ORIENTED_EDGE('',*,*,#8425,.F.);
#11488=ORIENTED_EDGE('',*,*,#8430,.F.);
#11489=ORIENTED_EDGE('',*,*,#8431,.T.);
#11490=ORIENTED_EDGE('',*,*,#8432,.F.);
#11491=ORIENTED_EDGE('',*,*,#8428,.F.);
#11492=ORIENTED_EDGE('',*,*,#8433,.F.);
#11493=ORIENTED_EDGE('',*,*,#8414,.T.);
#11494=ORIENTED_EDGE('',*,*,#8434,.F.);
#11495=ORIENTED_EDGE('',*,*,#8431,.F.);
#11496=ORIENTED_EDGE('',*,*,#8435,.F.);
#11497=ORIENTED_EDGE('',*,*,#8436,.T.);
#11498=ORIENTED_EDGE('',*,*,#8437,.F.);
#11499=ORIENTED_EDGE('',*,*,#8438,.F.);
#11500=ORIENTED_EDGE('',*,*,#8439,.F.);
#11501=ORIENTED_EDGE('',*,*,#8440,.T.);
#11502=ORIENTED_EDGE('',*,*,#8441,.F.);
#11503=ORIENTED_EDGE('',*,*,#8436,.F.);
#11504=ORIENTED_EDGE('',*,*,#8442,.F.);
#11505=ORIENTED_EDGE('',*,*,#8443,.T.);
#11506=ORIENTED_EDGE('',*,*,#8444,.F.);
#11507=ORIENTED_EDGE('',*,*,#8440,.F.);
#11508=ORIENTED_EDGE('',*,*,#8445,.F.);
#11509=ORIENTED_EDGE('',*,*,#8446,.T.);
#11510=ORIENTED_EDGE('',*,*,#8447,.F.);
#11511=ORIENTED_EDGE('',*,*,#8443,.F.);
#11512=ORIENTED_EDGE('',*,*,#8448,.F.);
#11513=ORIENTED_EDGE('',*,*,#8449,.T.);
#11514=ORIENTED_EDGE('',*,*,#8450,.F.);
#11515=ORIENTED_EDGE('',*,*,#8446,.F.);
#11516=ORIENTED_EDGE('',*,*,#8451,.F.);
#11517=ORIENTED_EDGE('',*,*,#8452,.T.);
#11518=ORIENTED_EDGE('',*,*,#8453,.F.);
#11519=ORIENTED_EDGE('',*,*,#8449,.F.);
#11520=ORIENTED_EDGE('',*,*,#8454,.F.);
#11521=ORIENTED_EDGE('',*,*,#8455,.T.);
#11522=ORIENTED_EDGE('',*,*,#8456,.F.);
#11523=ORIENTED_EDGE('',*,*,#8452,.F.);
#11524=ORIENTED_EDGE('',*,*,#8457,.F.);
#11525=ORIENTED_EDGE('',*,*,#8438,.T.);
#11526=ORIENTED_EDGE('',*,*,#8458,.F.);
#11527=ORIENTED_EDGE('',*,*,#8455,.F.);
#11528=ORIENTED_EDGE('',*,*,#8459,.F.);
#11529=ORIENTED_EDGE('',*,*,#8460,.T.);
#11530=ORIENTED_EDGE('',*,*,#8461,.F.);
#11531=ORIENTED_EDGE('',*,*,#8462,.F.);
#11532=ORIENTED_EDGE('',*,*,#8463,.F.);
#11533=ORIENTED_EDGE('',*,*,#8464,.T.);
#11534=ORIENTED_EDGE('',*,*,#8465,.F.);
#11535=ORIENTED_EDGE('',*,*,#8460,.F.);
#11536=ORIENTED_EDGE('',*,*,#8466,.F.);
#11537=ORIENTED_EDGE('',*,*,#8467,.T.);
#11538=ORIENTED_EDGE('',*,*,#8468,.F.);
#11539=ORIENTED_EDGE('',*,*,#8464,.F.);
#11540=ORIENTED_EDGE('',*,*,#8469,.F.);
#11541=ORIENTED_EDGE('',*,*,#8470,.T.);
#11542=ORIENTED_EDGE('',*,*,#8471,.F.);
#11543=ORIENTED_EDGE('',*,*,#8467,.F.);
#11544=ORIENTED_EDGE('',*,*,#8472,.F.);
#11545=ORIENTED_EDGE('',*,*,#8473,.T.);
#11546=ORIENTED_EDGE('',*,*,#8474,.F.);
#11547=ORIENTED_EDGE('',*,*,#8470,.F.);
#11548=ORIENTED_EDGE('',*,*,#8475,.F.);
#11549=ORIENTED_EDGE('',*,*,#8476,.T.);
#11550=ORIENTED_EDGE('',*,*,#8477,.F.);
#11551=ORIENTED_EDGE('',*,*,#8473,.F.);
#11552=ORIENTED_EDGE('',*,*,#8478,.F.);
#11553=ORIENTED_EDGE('',*,*,#8479,.T.);
#11554=ORIENTED_EDGE('',*,*,#8480,.F.);
#11555=ORIENTED_EDGE('',*,*,#8476,.F.);
#11556=ORIENTED_EDGE('',*,*,#8481,.F.);
#11557=ORIENTED_EDGE('',*,*,#8462,.T.);
#11558=ORIENTED_EDGE('',*,*,#8482,.F.);
#11559=ORIENTED_EDGE('',*,*,#8479,.F.);
#11560=ORIENTED_EDGE('',*,*,#8483,.F.);
#11561=ORIENTED_EDGE('',*,*,#8484,.T.);
#11562=ORIENTED_EDGE('',*,*,#8485,.F.);
#11563=ORIENTED_EDGE('',*,*,#8486,.F.);
#11564=ORIENTED_EDGE('',*,*,#8487,.F.);
#11565=ORIENTED_EDGE('',*,*,#8488,.T.);
#11566=ORIENTED_EDGE('',*,*,#8489,.F.);
#11567=ORIENTED_EDGE('',*,*,#8484,.F.);
#11568=ORIENTED_EDGE('',*,*,#8490,.F.);
#11569=ORIENTED_EDGE('',*,*,#8491,.T.);
#11570=ORIENTED_EDGE('',*,*,#8492,.F.);
#11571=ORIENTED_EDGE('',*,*,#8488,.F.);
#11572=ORIENTED_EDGE('',*,*,#8493,.F.);
#11573=ORIENTED_EDGE('',*,*,#8494,.T.);
#11574=ORIENTED_EDGE('',*,*,#8495,.F.);
#11575=ORIENTED_EDGE('',*,*,#8491,.F.);
#11576=ORIENTED_EDGE('',*,*,#8496,.F.);
#11577=ORIENTED_EDGE('',*,*,#8497,.T.);
#11578=ORIENTED_EDGE('',*,*,#8498,.F.);
#11579=ORIENTED_EDGE('',*,*,#8494,.F.);
#11580=ORIENTED_EDGE('',*,*,#8499,.F.);
#11581=ORIENTED_EDGE('',*,*,#8500,.T.);
#11582=ORIENTED_EDGE('',*,*,#8501,.F.);
#11583=ORIENTED_EDGE('',*,*,#8497,.F.);
#11584=ORIENTED_EDGE('',*,*,#8502,.F.);
#11585=ORIENTED_EDGE('',*,*,#8503,.T.);
#11586=ORIENTED_EDGE('',*,*,#8504,.F.);
#11587=ORIENTED_EDGE('',*,*,#8500,.F.);
#11588=ORIENTED_EDGE('',*,*,#8505,.F.);
#11589=ORIENTED_EDGE('',*,*,#8486,.T.);
#11590=ORIENTED_EDGE('',*,*,#8506,.F.);
#11591=ORIENTED_EDGE('',*,*,#8503,.F.);
#11592=ORIENTED_EDGE('',*,*,#8507,.F.);
#11593=ORIENTED_EDGE('',*,*,#8508,.T.);
#11594=ORIENTED_EDGE('',*,*,#8509,.F.);
#11595=ORIENTED_EDGE('',*,*,#8510,.F.);
#11596=ORIENTED_EDGE('',*,*,#8511,.F.);
#11597=ORIENTED_EDGE('',*,*,#8512,.T.);
#11598=ORIENTED_EDGE('',*,*,#8513,.F.);
#11599=ORIENTED_EDGE('',*,*,#8508,.F.);
#11600=ORIENTED_EDGE('',*,*,#8514,.F.);
#11601=ORIENTED_EDGE('',*,*,#8515,.T.);
#11602=ORIENTED_EDGE('',*,*,#8516,.F.);
#11603=ORIENTED_EDGE('',*,*,#8512,.F.);
#11604=ORIENTED_EDGE('',*,*,#8517,.F.);
#11605=ORIENTED_EDGE('',*,*,#8518,.T.);
#11606=ORIENTED_EDGE('',*,*,#8519,.F.);
#11607=ORIENTED_EDGE('',*,*,#8515,.F.);
#11608=ORIENTED_EDGE('',*,*,#8520,.F.);
#11609=ORIENTED_EDGE('',*,*,#8521,.T.);
#11610=ORIENTED_EDGE('',*,*,#8522,.F.);
#11611=ORIENTED_EDGE('',*,*,#8518,.F.);
#11612=ORIENTED_EDGE('',*,*,#8523,.F.);
#11613=ORIENTED_EDGE('',*,*,#8524,.T.);
#11614=ORIENTED_EDGE('',*,*,#8525,.F.);
#11615=ORIENTED_EDGE('',*,*,#8521,.F.);
#11616=ORIENTED_EDGE('',*,*,#8526,.F.);
#11617=ORIENTED_EDGE('',*,*,#8527,.T.);
#11618=ORIENTED_EDGE('',*,*,#8528,.F.);
#11619=ORIENTED_EDGE('',*,*,#8524,.F.);
#11620=ORIENTED_EDGE('',*,*,#8529,.F.);
#11621=ORIENTED_EDGE('',*,*,#8510,.T.);
#11622=ORIENTED_EDGE('',*,*,#8530,.F.);
#11623=ORIENTED_EDGE('',*,*,#8527,.F.);
#11624=ORIENTED_EDGE('',*,*,#8531,.F.);
#11625=ORIENTED_EDGE('',*,*,#8532,.T.);
#11626=ORIENTED_EDGE('',*,*,#8533,.F.);
#11627=ORIENTED_EDGE('',*,*,#8534,.F.);
#11628=ORIENTED_EDGE('',*,*,#8535,.F.);
#11629=ORIENTED_EDGE('',*,*,#8536,.T.);
#11630=ORIENTED_EDGE('',*,*,#8537,.F.);
#11631=ORIENTED_EDGE('',*,*,#8532,.F.);
#11632=ORIENTED_EDGE('',*,*,#8538,.F.);
#11633=ORIENTED_EDGE('',*,*,#8539,.T.);
#11634=ORIENTED_EDGE('',*,*,#8540,.F.);
#11635=ORIENTED_EDGE('',*,*,#8536,.F.);
#11636=ORIENTED_EDGE('',*,*,#8541,.F.);
#11637=ORIENTED_EDGE('',*,*,#8542,.T.);
#11638=ORIENTED_EDGE('',*,*,#8543,.F.);
#11639=ORIENTED_EDGE('',*,*,#8539,.F.);
#11640=ORIENTED_EDGE('',*,*,#8544,.F.);
#11641=ORIENTED_EDGE('',*,*,#8545,.T.);
#11642=ORIENTED_EDGE('',*,*,#8546,.F.);
#11643=ORIENTED_EDGE('',*,*,#8542,.F.);
#11644=ORIENTED_EDGE('',*,*,#8547,.F.);
#11645=ORIENTED_EDGE('',*,*,#8548,.T.);
#11646=ORIENTED_EDGE('',*,*,#8549,.F.);
#11647=ORIENTED_EDGE('',*,*,#8545,.F.);
#11648=ORIENTED_EDGE('',*,*,#8550,.F.);
#11649=ORIENTED_EDGE('',*,*,#8551,.T.);
#11650=ORIENTED_EDGE('',*,*,#8552,.F.);
#11651=ORIENTED_EDGE('',*,*,#8548,.F.);
#11652=ORIENTED_EDGE('',*,*,#8553,.F.);
#11653=ORIENTED_EDGE('',*,*,#8534,.T.);
#11654=ORIENTED_EDGE('',*,*,#8554,.F.);
#11655=ORIENTED_EDGE('',*,*,#8551,.F.);
#11656=ORIENTED_EDGE('',*,*,#8555,.F.);
#11657=ORIENTED_EDGE('',*,*,#8556,.T.);
#11658=ORIENTED_EDGE('',*,*,#8557,.F.);
#11659=ORIENTED_EDGE('',*,*,#8558,.F.);
#11660=ORIENTED_EDGE('',*,*,#8559,.F.);
#11661=ORIENTED_EDGE('',*,*,#8560,.T.);
#11662=ORIENTED_EDGE('',*,*,#8561,.F.);
#11663=ORIENTED_EDGE('',*,*,#8556,.F.);
#11664=ORIENTED_EDGE('',*,*,#8562,.F.);
#11665=ORIENTED_EDGE('',*,*,#8563,.T.);
#11666=ORIENTED_EDGE('',*,*,#8564,.F.);
#11667=ORIENTED_EDGE('',*,*,#8560,.F.);
#11668=ORIENTED_EDGE('',*,*,#8565,.F.);
#11669=ORIENTED_EDGE('',*,*,#8566,.T.);
#11670=ORIENTED_EDGE('',*,*,#8567,.F.);
#11671=ORIENTED_EDGE('',*,*,#8563,.F.);
#11672=ORIENTED_EDGE('',*,*,#8568,.F.);
#11673=ORIENTED_EDGE('',*,*,#8569,.T.);
#11674=ORIENTED_EDGE('',*,*,#8570,.F.);
#11675=ORIENTED_EDGE('',*,*,#8566,.F.);
#11676=ORIENTED_EDGE('',*,*,#8571,.F.);
#11677=ORIENTED_EDGE('',*,*,#8572,.T.);
#11678=ORIENTED_EDGE('',*,*,#8573,.F.);
#11679=ORIENTED_EDGE('',*,*,#8569,.F.);
#11680=ORIENTED_EDGE('',*,*,#8574,.F.);
#11681=ORIENTED_EDGE('',*,*,#8575,.T.);
#11682=ORIENTED_EDGE('',*,*,#8576,.F.);
#11683=ORIENTED_EDGE('',*,*,#8572,.F.);
#11684=ORIENTED_EDGE('',*,*,#8577,.F.);
#11685=ORIENTED_EDGE('',*,*,#8558,.T.);
#11686=ORIENTED_EDGE('',*,*,#8578,.F.);
#11687=ORIENTED_EDGE('',*,*,#8575,.F.);
#11688=ORIENTED_EDGE('',*,*,#8579,.F.);
#11689=ORIENTED_EDGE('',*,*,#8580,.T.);
#11690=ORIENTED_EDGE('',*,*,#8581,.F.);
#11691=ORIENTED_EDGE('',*,*,#8582,.F.);
#11692=ORIENTED_EDGE('',*,*,#8583,.F.);
#11693=ORIENTED_EDGE('',*,*,#8584,.T.);
#11694=ORIENTED_EDGE('',*,*,#8585,.F.);
#11695=ORIENTED_EDGE('',*,*,#8580,.F.);
#11696=ORIENTED_EDGE('',*,*,#8586,.F.);
#11697=ORIENTED_EDGE('',*,*,#8587,.T.);
#11698=ORIENTED_EDGE('',*,*,#8588,.F.);
#11699=ORIENTED_EDGE('',*,*,#8584,.F.);
#11700=ORIENTED_EDGE('',*,*,#8589,.F.);
#11701=ORIENTED_EDGE('',*,*,#8590,.T.);
#11702=ORIENTED_EDGE('',*,*,#8591,.F.);
#11703=ORIENTED_EDGE('',*,*,#8587,.F.);
#11704=ORIENTED_EDGE('',*,*,#8592,.F.);
#11705=ORIENTED_EDGE('',*,*,#8593,.T.);
#11706=ORIENTED_EDGE('',*,*,#8594,.F.);
#11707=ORIENTED_EDGE('',*,*,#8590,.F.);
#11708=ORIENTED_EDGE('',*,*,#8595,.F.);
#11709=ORIENTED_EDGE('',*,*,#8596,.T.);
#11710=ORIENTED_EDGE('',*,*,#8597,.F.);
#11711=ORIENTED_EDGE('',*,*,#8593,.F.);
#11712=ORIENTED_EDGE('',*,*,#8598,.F.);
#11713=ORIENTED_EDGE('',*,*,#8599,.T.);
#11714=ORIENTED_EDGE('',*,*,#8600,.F.);
#11715=ORIENTED_EDGE('',*,*,#8596,.F.);
#11716=ORIENTED_EDGE('',*,*,#8601,.F.);
#11717=ORIENTED_EDGE('',*,*,#8582,.T.);
#11718=ORIENTED_EDGE('',*,*,#8602,.F.);
#11719=ORIENTED_EDGE('',*,*,#8599,.F.);
#11720=ORIENTED_EDGE('',*,*,#8603,.F.);
#11721=ORIENTED_EDGE('',*,*,#8604,.T.);
#11722=ORIENTED_EDGE('',*,*,#8605,.F.);
#11723=ORIENTED_EDGE('',*,*,#8606,.F.);
#11724=ORIENTED_EDGE('',*,*,#8607,.F.);
#11725=ORIENTED_EDGE('',*,*,#8608,.T.);
#11726=ORIENTED_EDGE('',*,*,#8609,.F.);
#11727=ORIENTED_EDGE('',*,*,#8604,.F.);
#11728=ORIENTED_EDGE('',*,*,#8610,.F.);
#11729=ORIENTED_EDGE('',*,*,#8611,.T.);
#11730=ORIENTED_EDGE('',*,*,#8612,.F.);
#11731=ORIENTED_EDGE('',*,*,#8608,.F.);
#11732=ORIENTED_EDGE('',*,*,#8613,.F.);
#11733=ORIENTED_EDGE('',*,*,#8614,.T.);
#11734=ORIENTED_EDGE('',*,*,#8615,.F.);
#11735=ORIENTED_EDGE('',*,*,#8611,.F.);
#11736=ORIENTED_EDGE('',*,*,#8616,.F.);
#11737=ORIENTED_EDGE('',*,*,#8617,.T.);
#11738=ORIENTED_EDGE('',*,*,#8618,.F.);
#11739=ORIENTED_EDGE('',*,*,#8614,.F.);
#11740=ORIENTED_EDGE('',*,*,#8619,.F.);
#11741=ORIENTED_EDGE('',*,*,#8620,.T.);
#11742=ORIENTED_EDGE('',*,*,#8621,.F.);
#11743=ORIENTED_EDGE('',*,*,#8617,.F.);
#11744=ORIENTED_EDGE('',*,*,#8622,.F.);
#11745=ORIENTED_EDGE('',*,*,#8623,.T.);
#11746=ORIENTED_EDGE('',*,*,#8624,.F.);
#11747=ORIENTED_EDGE('',*,*,#8620,.F.);
#11748=ORIENTED_EDGE('',*,*,#8625,.F.);
#11749=ORIENTED_EDGE('',*,*,#8606,.T.);
#11750=ORIENTED_EDGE('',*,*,#8626,.F.);
#11751=ORIENTED_EDGE('',*,*,#8623,.F.);
#11752=ORIENTED_EDGE('',*,*,#8627,.F.);
#11753=ORIENTED_EDGE('',*,*,#8628,.T.);
#11754=ORIENTED_EDGE('',*,*,#8629,.F.);
#11755=ORIENTED_EDGE('',*,*,#8630,.F.);
#11756=ORIENTED_EDGE('',*,*,#8631,.F.);
#11757=ORIENTED_EDGE('',*,*,#8632,.T.);
#11758=ORIENTED_EDGE('',*,*,#8633,.F.);
#11759=ORIENTED_EDGE('',*,*,#8628,.F.);
#11760=ORIENTED_EDGE('',*,*,#8634,.F.);
#11761=ORIENTED_EDGE('',*,*,#8635,.T.);
#11762=ORIENTED_EDGE('',*,*,#8636,.F.);
#11763=ORIENTED_EDGE('',*,*,#8632,.F.);
#11764=ORIENTED_EDGE('',*,*,#8637,.F.);
#11765=ORIENTED_EDGE('',*,*,#8638,.T.);
#11766=ORIENTED_EDGE('',*,*,#8639,.F.);
#11767=ORIENTED_EDGE('',*,*,#8635,.F.);
#11768=ORIENTED_EDGE('',*,*,#8640,.F.);
#11769=ORIENTED_EDGE('',*,*,#8641,.T.);
#11770=ORIENTED_EDGE('',*,*,#8642,.F.);
#11771=ORIENTED_EDGE('',*,*,#8638,.F.);
#11772=ORIENTED_EDGE('',*,*,#8643,.F.);
#11773=ORIENTED_EDGE('',*,*,#8644,.T.);
#11774=ORIENTED_EDGE('',*,*,#8645,.F.);
#11775=ORIENTED_EDGE('',*,*,#8641,.F.);
#11776=ORIENTED_EDGE('',*,*,#8646,.F.);
#11777=ORIENTED_EDGE('',*,*,#8647,.T.);
#11778=ORIENTED_EDGE('',*,*,#8648,.F.);
#11779=ORIENTED_EDGE('',*,*,#8644,.F.);
#11780=ORIENTED_EDGE('',*,*,#8649,.F.);
#11781=ORIENTED_EDGE('',*,*,#8630,.T.);
#11782=ORIENTED_EDGE('',*,*,#8650,.F.);
#11783=ORIENTED_EDGE('',*,*,#8647,.F.);
#11784=ORIENTED_EDGE('',*,*,#8651,.F.);
#11785=ORIENTED_EDGE('',*,*,#8652,.T.);
#11786=ORIENTED_EDGE('',*,*,#8653,.F.);
#11787=ORIENTED_EDGE('',*,*,#8654,.F.);
#11788=ORIENTED_EDGE('',*,*,#8655,.F.);
#11789=ORIENTED_EDGE('',*,*,#8656,.T.);
#11790=ORIENTED_EDGE('',*,*,#8657,.F.);
#11791=ORIENTED_EDGE('',*,*,#8652,.F.);
#11792=ORIENTED_EDGE('',*,*,#8658,.F.);
#11793=ORIENTED_EDGE('',*,*,#8659,.T.);
#11794=ORIENTED_EDGE('',*,*,#8660,.F.);
#11795=ORIENTED_EDGE('',*,*,#8656,.F.);
#11796=ORIENTED_EDGE('',*,*,#8661,.F.);
#11797=ORIENTED_EDGE('',*,*,#8662,.T.);
#11798=ORIENTED_EDGE('',*,*,#8663,.F.);
#11799=ORIENTED_EDGE('',*,*,#8659,.F.);
#11800=ORIENTED_EDGE('',*,*,#8664,.F.);
#11801=ORIENTED_EDGE('',*,*,#8665,.T.);
#11802=ORIENTED_EDGE('',*,*,#8666,.F.);
#11803=ORIENTED_EDGE('',*,*,#8662,.F.);
#11804=ORIENTED_EDGE('',*,*,#8667,.F.);
#11805=ORIENTED_EDGE('',*,*,#8668,.T.);
#11806=ORIENTED_EDGE('',*,*,#8669,.F.);
#11807=ORIENTED_EDGE('',*,*,#8665,.F.);
#11808=ORIENTED_EDGE('',*,*,#8670,.F.);
#11809=ORIENTED_EDGE('',*,*,#8671,.T.);
#11810=ORIENTED_EDGE('',*,*,#8672,.F.);
#11811=ORIENTED_EDGE('',*,*,#8668,.F.);
#11812=ORIENTED_EDGE('',*,*,#8673,.F.);
#11813=ORIENTED_EDGE('',*,*,#8654,.T.);
#11814=ORIENTED_EDGE('',*,*,#8674,.F.);
#11815=ORIENTED_EDGE('',*,*,#8671,.F.);
#11816=ORIENTED_EDGE('',*,*,#8675,.F.);
#11817=ORIENTED_EDGE('',*,*,#8676,.T.);
#11818=ORIENTED_EDGE('',*,*,#8677,.F.);
#11819=ORIENTED_EDGE('',*,*,#8678,.F.);
#11820=ORIENTED_EDGE('',*,*,#8679,.F.);
#11821=ORIENTED_EDGE('',*,*,#8680,.T.);
#11822=ORIENTED_EDGE('',*,*,#8681,.F.);
#11823=ORIENTED_EDGE('',*,*,#8676,.F.);
#11824=ORIENTED_EDGE('',*,*,#8682,.F.);
#11825=ORIENTED_EDGE('',*,*,#8683,.T.);
#11826=ORIENTED_EDGE('',*,*,#8684,.F.);
#11827=ORIENTED_EDGE('',*,*,#8680,.F.);
#11828=ORIENTED_EDGE('',*,*,#8685,.F.);
#11829=ORIENTED_EDGE('',*,*,#8686,.T.);
#11830=ORIENTED_EDGE('',*,*,#8687,.F.);
#11831=ORIENTED_EDGE('',*,*,#8683,.F.);
#11832=ORIENTED_EDGE('',*,*,#8688,.F.);
#11833=ORIENTED_EDGE('',*,*,#8689,.T.);
#11834=ORIENTED_EDGE('',*,*,#8690,.F.);
#11835=ORIENTED_EDGE('',*,*,#8686,.F.);
#11836=ORIENTED_EDGE('',*,*,#8691,.F.);
#11837=ORIENTED_EDGE('',*,*,#8692,.T.);
#11838=ORIENTED_EDGE('',*,*,#8693,.F.);
#11839=ORIENTED_EDGE('',*,*,#8689,.F.);
#11840=ORIENTED_EDGE('',*,*,#8694,.F.);
#11841=ORIENTED_EDGE('',*,*,#8695,.T.);
#11842=ORIENTED_EDGE('',*,*,#8696,.F.);
#11843=ORIENTED_EDGE('',*,*,#8692,.F.);
#11844=ORIENTED_EDGE('',*,*,#8697,.F.);
#11845=ORIENTED_EDGE('',*,*,#8678,.T.);
#11846=ORIENTED_EDGE('',*,*,#8698,.F.);
#11847=ORIENTED_EDGE('',*,*,#8695,.F.);
#11848=ORIENTED_EDGE('',*,*,#8699,.F.);
#11849=ORIENTED_EDGE('',*,*,#8700,.T.);
#11850=ORIENTED_EDGE('',*,*,#8701,.F.);
#11851=ORIENTED_EDGE('',*,*,#8702,.F.);
#11852=ORIENTED_EDGE('',*,*,#8703,.F.);
#11853=ORIENTED_EDGE('',*,*,#8704,.T.);
#11854=ORIENTED_EDGE('',*,*,#8705,.F.);
#11855=ORIENTED_EDGE('',*,*,#8700,.F.);
#11856=ORIENTED_EDGE('',*,*,#8706,.F.);
#11857=ORIENTED_EDGE('',*,*,#8707,.T.);
#11858=ORIENTED_EDGE('',*,*,#8708,.F.);
#11859=ORIENTED_EDGE('',*,*,#8704,.F.);
#11860=ORIENTED_EDGE('',*,*,#8709,.F.);
#11861=ORIENTED_EDGE('',*,*,#8710,.T.);
#11862=ORIENTED_EDGE('',*,*,#8711,.F.);
#11863=ORIENTED_EDGE('',*,*,#8707,.F.);
#11864=ORIENTED_EDGE('',*,*,#8712,.F.);
#11865=ORIENTED_EDGE('',*,*,#8713,.T.);
#11866=ORIENTED_EDGE('',*,*,#8714,.F.);
#11867=ORIENTED_EDGE('',*,*,#8710,.F.);
#11868=ORIENTED_EDGE('',*,*,#8715,.F.);
#11869=ORIENTED_EDGE('',*,*,#8716,.T.);
#11870=ORIENTED_EDGE('',*,*,#8717,.F.);
#11871=ORIENTED_EDGE('',*,*,#8713,.F.);
#11872=ORIENTED_EDGE('',*,*,#8718,.F.);
#11873=ORIENTED_EDGE('',*,*,#8719,.T.);
#11874=ORIENTED_EDGE('',*,*,#8720,.F.);
#11875=ORIENTED_EDGE('',*,*,#8716,.F.);
#11876=ORIENTED_EDGE('',*,*,#8721,.F.);
#11877=ORIENTED_EDGE('',*,*,#8702,.T.);
#11878=ORIENTED_EDGE('',*,*,#8722,.F.);
#11879=ORIENTED_EDGE('',*,*,#8719,.F.);
#11880=ORIENTED_EDGE('',*,*,#8723,.T.);
#11881=ORIENTED_EDGE('',*,*,#8724,.T.);
#11882=ORIENTED_EDGE('',*,*,#8725,.F.);
#11883=ORIENTED_EDGE('',*,*,#8726,.F.);
#11884=ORIENTED_EDGE('',*,*,#8727,.T.);
#11885=ORIENTED_EDGE('',*,*,#8726,.T.);
#11886=ORIENTED_EDGE('',*,*,#8728,.F.);
#11887=ORIENTED_EDGE('',*,*,#8729,.F.);
#11888=ORIENTED_EDGE('',*,*,#8730,.T.);
#11889=ORIENTED_EDGE('',*,*,#8729,.T.);
#11890=ORIENTED_EDGE('',*,*,#8731,.F.);
#11891=ORIENTED_EDGE('',*,*,#8732,.F.);
#11892=ORIENTED_EDGE('',*,*,#8733,.T.);
#11893=ORIENTED_EDGE('',*,*,#8732,.T.);
#11894=ORIENTED_EDGE('',*,*,#8734,.F.);
#11895=ORIENTED_EDGE('',*,*,#8735,.F.);
#11896=ORIENTED_EDGE('',*,*,#8736,.T.);
#11897=ORIENTED_EDGE('',*,*,#8735,.T.);
#11898=ORIENTED_EDGE('',*,*,#8737,.F.);
#11899=ORIENTED_EDGE('',*,*,#8738,.F.);
#11900=ORIENTED_EDGE('',*,*,#8739,.T.);
#11901=ORIENTED_EDGE('',*,*,#8738,.T.);
#11902=ORIENTED_EDGE('',*,*,#8740,.F.);
#11903=ORIENTED_EDGE('',*,*,#8741,.F.);
#11904=ORIENTED_EDGE('',*,*,#8742,.T.);
#11905=ORIENTED_EDGE('',*,*,#8741,.T.);
#11906=ORIENTED_EDGE('',*,*,#8743,.F.);
#11907=ORIENTED_EDGE('',*,*,#8744,.F.);
#11908=ORIENTED_EDGE('',*,*,#8745,.T.);
#11909=ORIENTED_EDGE('',*,*,#8744,.T.);
#11910=ORIENTED_EDGE('',*,*,#8746,.F.);
#11911=ORIENTED_EDGE('',*,*,#8724,.F.);
#11912=ORIENTED_EDGE('',*,*,#8746,.T.);
#11913=ORIENTED_EDGE('',*,*,#8743,.T.);
#11914=ORIENTED_EDGE('',*,*,#8740,.T.);
#11915=ORIENTED_EDGE('',*,*,#8737,.T.);
#11916=ORIENTED_EDGE('',*,*,#8734,.T.);
#11917=ORIENTED_EDGE('',*,*,#8731,.T.);
#11918=ORIENTED_EDGE('',*,*,#8728,.T.);
#11919=ORIENTED_EDGE('',*,*,#8725,.T.);
#11920=ORIENTED_EDGE('',*,*,#8389,.T.);
#11921=ORIENTED_EDGE('',*,*,#8393,.T.);
#11922=ORIENTED_EDGE('',*,*,#8396,.T.);
#11923=ORIENTED_EDGE('',*,*,#8399,.T.);
#11924=ORIENTED_EDGE('',*,*,#8402,.T.);
#11925=ORIENTED_EDGE('',*,*,#8405,.T.);
#11926=ORIENTED_EDGE('',*,*,#8408,.T.);
#11927=ORIENTED_EDGE('',*,*,#8410,.T.);
#11928=ORIENTED_EDGE('',*,*,#8701,.T.);
#11929=ORIENTED_EDGE('',*,*,#8705,.T.);
#11930=ORIENTED_EDGE('',*,*,#8708,.T.);
#11931=ORIENTED_EDGE('',*,*,#8711,.T.);
#11932=ORIENTED_EDGE('',*,*,#8714,.T.);
#11933=ORIENTED_EDGE('',*,*,#8717,.T.);
#11934=ORIENTED_EDGE('',*,*,#8720,.T.);
#11935=ORIENTED_EDGE('',*,*,#8722,.T.);
#11936=ORIENTED_EDGE('',*,*,#8677,.T.);
#11937=ORIENTED_EDGE('',*,*,#8681,.T.);
#11938=ORIENTED_EDGE('',*,*,#8684,.T.);
#11939=ORIENTED_EDGE('',*,*,#8687,.T.);
#11940=ORIENTED_EDGE('',*,*,#8690,.T.);
#11941=ORIENTED_EDGE('',*,*,#8693,.T.);
#11942=ORIENTED_EDGE('',*,*,#8696,.T.);
#11943=ORIENTED_EDGE('',*,*,#8698,.T.);
#11944=ORIENTED_EDGE('',*,*,#8653,.T.);
#11945=ORIENTED_EDGE('',*,*,#8657,.T.);
#11946=ORIENTED_EDGE('',*,*,#8660,.T.);
#11947=ORIENTED_EDGE('',*,*,#8663,.T.);
#11948=ORIENTED_EDGE('',*,*,#8666,.T.);
#11949=ORIENTED_EDGE('',*,*,#8669,.T.);
#11950=ORIENTED_EDGE('',*,*,#8672,.T.);
#11951=ORIENTED_EDGE('',*,*,#8674,.T.);
#11952=ORIENTED_EDGE('',*,*,#8629,.T.);
#11953=ORIENTED_EDGE('',*,*,#8633,.T.);
#11954=ORIENTED_EDGE('',*,*,#8636,.T.);
#11955=ORIENTED_EDGE('',*,*,#8639,.T.);
#11956=ORIENTED_EDGE('',*,*,#8642,.T.);
#11957=ORIENTED_EDGE('',*,*,#8645,.T.);
#11958=ORIENTED_EDGE('',*,*,#8648,.T.);
#11959=ORIENTED_EDGE('',*,*,#8650,.T.);
#11960=ORIENTED_EDGE('',*,*,#8605,.T.);
#11961=ORIENTED_EDGE('',*,*,#8609,.T.);
#11962=ORIENTED_EDGE('',*,*,#8612,.T.);
#11963=ORIENTED_EDGE('',*,*,#8615,.T.);
#11964=ORIENTED_EDGE('',*,*,#8618,.T.);
#11965=ORIENTED_EDGE('',*,*,#8621,.T.);
#11966=ORIENTED_EDGE('',*,*,#8624,.T.);
#11967=ORIENTED_EDGE('',*,*,#8626,.T.);
#11968=ORIENTED_EDGE('',*,*,#8581,.T.);
#11969=ORIENTED_EDGE('',*,*,#8585,.T.);
#11970=ORIENTED_EDGE('',*,*,#8588,.T.);
#11971=ORIENTED_EDGE('',*,*,#8591,.T.);
#11972=ORIENTED_EDGE('',*,*,#8594,.T.);
#11973=ORIENTED_EDGE('',*,*,#8597,.T.);
#11974=ORIENTED_EDGE('',*,*,#8600,.T.);
#11975=ORIENTED_EDGE('',*,*,#8602,.T.);
#11976=ORIENTED_EDGE('',*,*,#8557,.T.);
#11977=ORIENTED_EDGE('',*,*,#8561,.T.);
#11978=ORIENTED_EDGE('',*,*,#8564,.T.);
#11979=ORIENTED_EDGE('',*,*,#8567,.T.);
#11980=ORIENTED_EDGE('',*,*,#8570,.T.);
#11981=ORIENTED_EDGE('',*,*,#8573,.T.);
#11982=ORIENTED_EDGE('',*,*,#8576,.T.);
#11983=ORIENTED_EDGE('',*,*,#8578,.T.);
#11984=ORIENTED_EDGE('',*,*,#8533,.T.);
#11985=ORIENTED_EDGE('',*,*,#8537,.T.);
#11986=ORIENTED_EDGE('',*,*,#8540,.T.);
#11987=ORIENTED_EDGE('',*,*,#8543,.T.);
#11988=ORIENTED_EDGE('',*,*,#8546,.T.);
#11989=ORIENTED_EDGE('',*,*,#8549,.T.);
#11990=ORIENTED_EDGE('',*,*,#8552,.T.);
#11991=ORIENTED_EDGE('',*,*,#8554,.T.);
#11992=ORIENTED_EDGE('',*,*,#8509,.T.);
#11993=ORIENTED_EDGE('',*,*,#8513,.T.);
#11994=ORIENTED_EDGE('',*,*,#8516,.T.);
#11995=ORIENTED_EDGE('',*,*,#8519,.T.);
#11996=ORIENTED_EDGE('',*,*,#8522,.T.);
#11997=ORIENTED_EDGE('',*,*,#8525,.T.);
#11998=ORIENTED_EDGE('',*,*,#8528,.T.);
#11999=ORIENTED_EDGE('',*,*,#8530,.T.);
#12000=ORIENTED_EDGE('',*,*,#8485,.T.);
#12001=ORIENTED_EDGE('',*,*,#8489,.T.);
#12002=ORIENTED_EDGE('',*,*,#8492,.T.);
#12003=ORIENTED_EDGE('',*,*,#8495,.T.);
#12004=ORIENTED_EDGE('',*,*,#8498,.T.);
#12005=ORIENTED_EDGE('',*,*,#8501,.T.);
#12006=ORIENTED_EDGE('',*,*,#8504,.T.);
#12007=ORIENTED_EDGE('',*,*,#8506,.T.);
#12008=ORIENTED_EDGE('',*,*,#8461,.T.);
#12009=ORIENTED_EDGE('',*,*,#8465,.T.);
#12010=ORIENTED_EDGE('',*,*,#8468,.T.);
#12011=ORIENTED_EDGE('',*,*,#8471,.T.);
#12012=ORIENTED_EDGE('',*,*,#8474,.T.);
#12013=ORIENTED_EDGE('',*,*,#8477,.T.);
#12014=ORIENTED_EDGE('',*,*,#8480,.T.);
#12015=ORIENTED_EDGE('',*,*,#8482,.T.);
#12016=ORIENTED_EDGE('',*,*,#8437,.T.);
#12017=ORIENTED_EDGE('',*,*,#8441,.T.);
#12018=ORIENTED_EDGE('',*,*,#8444,.T.);
#12019=ORIENTED_EDGE('',*,*,#8447,.T.);
#12020=ORIENTED_EDGE('',*,*,#8450,.T.);
#12021=ORIENTED_EDGE('',*,*,#8453,.T.);
#12022=ORIENTED_EDGE('',*,*,#8456,.T.);
#12023=ORIENTED_EDGE('',*,*,#8458,.T.);
#12024=ORIENTED_EDGE('',*,*,#8413,.T.);
#12025=ORIENTED_EDGE('',*,*,#8417,.T.);
#12026=ORIENTED_EDGE('',*,*,#8420,.T.);
#12027=ORIENTED_EDGE('',*,*,#8423,.T.);
#12028=ORIENTED_EDGE('',*,*,#8426,.T.);
#12029=ORIENTED_EDGE('',*,*,#8429,.T.);
#12030=ORIENTED_EDGE('',*,*,#8432,.T.);
#12031=ORIENTED_EDGE('',*,*,#8434,.T.);
#12032=ORIENTED_EDGE('',*,*,#8365,.T.);
#12033=ORIENTED_EDGE('',*,*,#8369,.T.);
#12034=ORIENTED_EDGE('',*,*,#8372,.T.);
#12035=ORIENTED_EDGE('',*,*,#8375,.T.);
#12036=ORIENTED_EDGE('',*,*,#8378,.T.);
#12037=ORIENTED_EDGE('',*,*,#8381,.T.);
#12038=ORIENTED_EDGE('',*,*,#8384,.T.);
#12039=ORIENTED_EDGE('',*,*,#8386,.T.);
#12040=ORIENTED_EDGE('',*,*,#8745,.F.);
#12041=ORIENTED_EDGE('',*,*,#8723,.F.);
#12042=ORIENTED_EDGE('',*,*,#8727,.F.);
#12043=ORIENTED_EDGE('',*,*,#8730,.F.);
#12044=ORIENTED_EDGE('',*,*,#8733,.F.);
#12045=ORIENTED_EDGE('',*,*,#8736,.F.);
#12046=ORIENTED_EDGE('',*,*,#8739,.F.);
#12047=ORIENTED_EDGE('',*,*,#8742,.F.);
#12048=ORIENTED_EDGE('',*,*,#8387,.T.);
#12049=ORIENTED_EDGE('',*,*,#8409,.T.);
#12050=ORIENTED_EDGE('',*,*,#8406,.T.);
#12051=ORIENTED_EDGE('',*,*,#8403,.T.);
#12052=ORIENTED_EDGE('',*,*,#8400,.T.);
#12053=ORIENTED_EDGE('',*,*,#8397,.T.);
#12054=ORIENTED_EDGE('',*,*,#8394,.T.);
#12055=ORIENTED_EDGE('',*,*,#8391,.T.);
#12056=ORIENTED_EDGE('',*,*,#8699,.T.);
#12057=ORIENTED_EDGE('',*,*,#8721,.T.);
#12058=ORIENTED_EDGE('',*,*,#8718,.T.);
#12059=ORIENTED_EDGE('',*,*,#8715,.T.);
#12060=ORIENTED_EDGE('',*,*,#8712,.T.);
#12061=ORIENTED_EDGE('',*,*,#8709,.T.);
#12062=ORIENTED_EDGE('',*,*,#8706,.T.);
#12063=ORIENTED_EDGE('',*,*,#8703,.T.);
#12064=ORIENTED_EDGE('',*,*,#8675,.T.);
#12065=ORIENTED_EDGE('',*,*,#8697,.T.);
#12066=ORIENTED_EDGE('',*,*,#8694,.T.);
#12067=ORIENTED_EDGE('',*,*,#8691,.T.);
#12068=ORIENTED_EDGE('',*,*,#8688,.T.);
#12069=ORIENTED_EDGE('',*,*,#8685,.T.);
#12070=ORIENTED_EDGE('',*,*,#8682,.T.);
#12071=ORIENTED_EDGE('',*,*,#8679,.T.);
#12072=ORIENTED_EDGE('',*,*,#8651,.T.);
#12073=ORIENTED_EDGE('',*,*,#8673,.T.);
#12074=ORIENTED_EDGE('',*,*,#8670,.T.);
#12075=ORIENTED_EDGE('',*,*,#8667,.T.);
#12076=ORIENTED_EDGE('',*,*,#8664,.T.);
#12077=ORIENTED_EDGE('',*,*,#8661,.T.);
#12078=ORIENTED_EDGE('',*,*,#8658,.T.);
#12079=ORIENTED_EDGE('',*,*,#8655,.T.);
#12080=ORIENTED_EDGE('',*,*,#8627,.T.);
#12081=ORIENTED_EDGE('',*,*,#8649,.T.);
#12082=ORIENTED_EDGE('',*,*,#8646,.T.);
#12083=ORIENTED_EDGE('',*,*,#8643,.T.);
#12084=ORIENTED_EDGE('',*,*,#8640,.T.);
#12085=ORIENTED_EDGE('',*,*,#8637,.T.);
#12086=ORIENTED_EDGE('',*,*,#8634,.T.);
#12087=ORIENTED_EDGE('',*,*,#8631,.T.);
#12088=ORIENTED_EDGE('',*,*,#8603,.T.);
#12089=ORIENTED_EDGE('',*,*,#8625,.T.);
#12090=ORIENTED_EDGE('',*,*,#8622,.T.);
#12091=ORIENTED_EDGE('',*,*,#8619,.T.);
#12092=ORIENTED_EDGE('',*,*,#8616,.T.);
#12093=ORIENTED_EDGE('',*,*,#8613,.T.);
#12094=ORIENTED_EDGE('',*,*,#8610,.T.);
#12095=ORIENTED_EDGE('',*,*,#8607,.T.);
#12096=ORIENTED_EDGE('',*,*,#8579,.T.);
#12097=ORIENTED_EDGE('',*,*,#8601,.T.);
#12098=ORIENTED_EDGE('',*,*,#8598,.T.);
#12099=ORIENTED_EDGE('',*,*,#8595,.T.);
#12100=ORIENTED_EDGE('',*,*,#8592,.T.);
#12101=ORIENTED_EDGE('',*,*,#8589,.T.);
#12102=ORIENTED_EDGE('',*,*,#8586,.T.);
#12103=ORIENTED_EDGE('',*,*,#8583,.T.);
#12104=ORIENTED_EDGE('',*,*,#8555,.T.);
#12105=ORIENTED_EDGE('',*,*,#8577,.T.);
#12106=ORIENTED_EDGE('',*,*,#8574,.T.);
#12107=ORIENTED_EDGE('',*,*,#8571,.T.);
#12108=ORIENTED_EDGE('',*,*,#8568,.T.);
#12109=ORIENTED_EDGE('',*,*,#8565,.T.);
#12110=ORIENTED_EDGE('',*,*,#8562,.T.);
#12111=ORIENTED_EDGE('',*,*,#8559,.T.);
#12112=ORIENTED_EDGE('',*,*,#8531,.T.);
#12113=ORIENTED_EDGE('',*,*,#8553,.T.);
#12114=ORIENTED_EDGE('',*,*,#8550,.T.);
#12115=ORIENTED_EDGE('',*,*,#8547,.T.);
#12116=ORIENTED_EDGE('',*,*,#8544,.T.);
#12117=ORIENTED_EDGE('',*,*,#8541,.T.);
#12118=ORIENTED_EDGE('',*,*,#8538,.T.);
#12119=ORIENTED_EDGE('',*,*,#8535,.T.);
#12120=ORIENTED_EDGE('',*,*,#8507,.T.);
#12121=ORIENTED_EDGE('',*,*,#8529,.T.);
#12122=ORIENTED_EDGE('',*,*,#8526,.T.);
#12123=ORIENTED_EDGE('',*,*,#8523,.T.);
#12124=ORIENTED_EDGE('',*,*,#8520,.T.);
#12125=ORIENTED_EDGE('',*,*,#8517,.T.);
#12126=ORIENTED_EDGE('',*,*,#8514,.T.);
#12127=ORIENTED_EDGE('',*,*,#8511,.T.);
#12128=ORIENTED_EDGE('',*,*,#8483,.T.);
#12129=ORIENTED_EDGE('',*,*,#8505,.T.);
#12130=ORIENTED_EDGE('',*,*,#8502,.T.);
#12131=ORIENTED_EDGE('',*,*,#8499,.T.);
#12132=ORIENTED_EDGE('',*,*,#8496,.T.);
#12133=ORIENTED_EDGE('',*,*,#8493,.T.);
#12134=ORIENTED_EDGE('',*,*,#8490,.T.);
#12135=ORIENTED_EDGE('',*,*,#8487,.T.);
#12136=ORIENTED_EDGE('',*,*,#8459,.T.);
#12137=ORIENTED_EDGE('',*,*,#8481,.T.);
#12138=ORIENTED_EDGE('',*,*,#8478,.T.);
#12139=ORIENTED_EDGE('',*,*,#8475,.T.);
#12140=ORIENTED_EDGE('',*,*,#8472,.T.);
#12141=ORIENTED_EDGE('',*,*,#8469,.T.);
#12142=ORIENTED_EDGE('',*,*,#8466,.T.);
#12143=ORIENTED_EDGE('',*,*,#8463,.T.);
#12144=ORIENTED_EDGE('',*,*,#8435,.T.);
#12145=ORIENTED_EDGE('',*,*,#8457,.T.);
#12146=ORIENTED_EDGE('',*,*,#8454,.T.);
#12147=ORIENTED_EDGE('',*,*,#8451,.T.);
#12148=ORIENTED_EDGE('',*,*,#8448,.T.);
#12149=ORIENTED_EDGE('',*,*,#8445,.T.);
#12150=ORIENTED_EDGE('',*,*,#8442,.T.);
#12151=ORIENTED_EDGE('',*,*,#8439,.T.);
#12152=ORIENTED_EDGE('',*,*,#8411,.T.);
#12153=ORIENTED_EDGE('',*,*,#8433,.T.);
#12154=ORIENTED_EDGE('',*,*,#8430,.T.);
#12155=ORIENTED_EDGE('',*,*,#8427,.T.);
#12156=ORIENTED_EDGE('',*,*,#8424,.T.);
#12157=ORIENTED_EDGE('',*,*,#8421,.T.);
#12158=ORIENTED_EDGE('',*,*,#8418,.T.);
#12159=ORIENTED_EDGE('',*,*,#8415,.T.);
#12160=ORIENTED_EDGE('',*,*,#8363,.T.);
#12161=ORIENTED_EDGE('',*,*,#8385,.T.);
#12162=ORIENTED_EDGE('',*,*,#8382,.T.);
#12163=ORIENTED_EDGE('',*,*,#8379,.T.);
#12164=ORIENTED_EDGE('',*,*,#8376,.T.);
#12165=ORIENTED_EDGE('',*,*,#8373,.T.);
#12166=ORIENTED_EDGE('',*,*,#8370,.T.);
#12167=ORIENTED_EDGE('',*,*,#8367,.T.);
#14654=ADVANCED_FACE('',(#1919),#1362,.F.);
#14655=ADVANCED_FACE('',(#1920),#926,.F.);
#14656=ADVANCED_FACE('',(#1921),#1363,.F.);
#14657=ADVANCED_FACE('',(#1922),#927,.F.);
#14658=ADVANCED_FACE('',(#1923),#1364,.F.);
#14659=ADVANCED_FACE('',(#1924),#928,.F.);
#14660=ADVANCED_FACE('',(#1925),#1365,.F.);
#14661=ADVANCED_FACE('',(#1926),#929,.F.);
#14662=ADVANCED_FACE('',(#1927),#1366,.F.);
#14663=ADVANCED_FACE('',(#1928),#930,.F.);
#14664=ADVANCED_FACE('',(#1929),#1367,.F.);
#14665=ADVANCED_FACE('',(#1930),#931,.F.);
#14666=ADVANCED_FACE('',(#1931),#1368,.F.);
#14667=ADVANCED_FACE('',(#1932),#932,.F.);
#14668=ADVANCED_FACE('',(#1933),#1369,.F.);
#14669=ADVANCED_FACE('',(#1934),#933,.F.);
#14670=ADVANCED_FACE('',(#1935),#1370,.F.);
#14671=ADVANCED_FACE('',(#1936),#934,.F.);
#14672=ADVANCED_FACE('',(#1937),#1371,.F.);
#14673=ADVANCED_FACE('',(#1938),#935,.F.);
#14674=ADVANCED_FACE('',(#1939),#1372,.F.);
#14675=ADVANCED_FACE('',(#1940),#936,.F.);
#14676=ADVANCED_FACE('',(#1941),#1373,.F.);
#14677=ADVANCED_FACE('',(#1942),#937,.F.);
#14678=ADVANCED_FACE('',(#1943),#1374,.F.);
#14679=ADVANCED_FACE('',(#1944),#938,.F.);
#14680=ADVANCED_FACE('',(#1945),#1375,.F.);
#14681=ADVANCED_FACE('',(#1946),#939,.F.);
#14682=ADVANCED_FACE('',(#1947),#1376,.F.);
#14683=ADVANCED_FACE('',(#1948),#940,.F.);
#14684=ADVANCED_FACE('',(#1949),#1377,.F.);
#14685=ADVANCED_FACE('',(#1950),#941,.F.);
#14686=ADVANCED_FACE('',(#1951),#1378,.F.);
#14687=ADVANCED_FACE('',(#1952),#942,.F.);
#14688=ADVANCED_FACE('',(#1953),#1379,.F.);
#14689=ADVANCED_FACE('',(#1954),#943,.F.);
#14690=ADVANCED_FACE('',(#1955),#1380,.F.);
#14691=ADVANCED_FACE('',(#1956),#944,.F.);
#14692=ADVANCED_FACE('',(#1957),#1381,.F.);
#14693=ADVANCED_FACE('',(#1958),#945,.F.);
#14694=ADVANCED_FACE('',(#1959),#1382,.F.);
#14695=ADVANCED_FACE('',(#1960),#946,.F.);
#14696=ADVANCED_FACE('',(#1961),#1383,.F.);
#14697=ADVANCED_FACE('',(#1962),#947,.F.);
#14698=ADVANCED_FACE('',(#1963),#1384,.F.);
#14699=ADVANCED_FACE('',(#1964),#948,.F.);
#14700=ADVANCED_FACE('',(#1965),#1385,.F.);
#14701=ADVANCED_FACE('',(#1966),#949,.F.);
#14702=ADVANCED_FACE('',(#1967),#1386,.F.);
#14703=ADVANCED_FACE('',(#1968),#950,.F.);
#14704=ADVANCED_FACE('',(#1969),#1387,.F.);
#14705=ADVANCED_FACE('',(#1970),#951,.F.);
#14706=ADVANCED_FACE('',(#1971),#1388,.F.);
#14707=ADVANCED_FACE('',(#1972),#952,.F.);
#14708=ADVANCED_FACE('',(#1973),#1389,.F.);
#14709=ADVANCED_FACE('',(#1974),#953,.F.);
#14710=ADVANCED_FACE('',(#1975),#1390,.F.);
#14711=ADVANCED_FACE('',(#1976),#954,.F.);
#14712=ADVANCED_FACE('',(#1977),#1391,.F.);
#14713=ADVANCED_FACE('',(#1978),#955,.F.);
#14714=ADVANCED_FACE('',(#1979),#1392,.F.);
#14715=ADVANCED_FACE('',(#1980),#956,.F.);
#14716=ADVANCED_FACE('',(#1981),#1393,.F.);
#14717=ADVANCED_FACE('',(#1982),#957,.F.);
#14718=ADVANCED_FACE('',(#1983),#1394,.F.);
#14719=ADVANCED_FACE('',(#1984),#958,.F.);
#14720=ADVANCED_FACE('',(#1985),#1395,.F.);
#14721=ADVANCED_FACE('',(#1986),#959,.F.);
#14722=ADVANCED_FACE('',(#1987),#1396,.F.);
#14723=ADVANCED_FACE('',(#1988),#960,.F.);
#14724=ADVANCED_FACE('',(#1989),#1397,.F.);
#14725=ADVANCED_FACE('',(#1990),#961,.F.);
#14726=ADVANCED_FACE('',(#1991),#1398,.F.);
#14727=ADVANCED_FACE('',(#1992),#962,.F.);
#14728=ADVANCED_FACE('',(#1993),#1399,.F.);
#14729=ADVANCED_FACE('',(#1994),#963,.F.);
#14730=ADVANCED_FACE('',(#1995),#1400,.F.);
#14731=ADVANCED_FACE('',(#1996),#964,.F.);
#14732=ADVANCED_FACE('',(#1997),#1401,.F.);
#14733=ADVANCED_FACE('',(#1998),#965,.F.);
#14734=ADVANCED_FACE('',(#1999),#1402,.F.);
#14735=ADVANCED_FACE('',(#2000),#966,.F.);
#14736=ADVANCED_FACE('',(#2001),#1403,.F.);
#14737=ADVANCED_FACE('',(#2002),#967,.F.);
#14738=ADVANCED_FACE('',(#2003),#1404,.F.);
#14739=ADVANCED_FACE('',(#2004),#968,.F.);
#14740=ADVANCED_FACE('',(#2005),#1405,.F.);
#14741=ADVANCED_FACE('',(#2006),#969,.F.);
#14742=ADVANCED_FACE('',(#2007),#1406,.F.);
#14743=ADVANCED_FACE('',(#2008),#970,.F.);
#14744=ADVANCED_FACE('',(#2009),#1407,.F.);
#14745=ADVANCED_FACE('',(#2010),#971,.F.);
#14746=ADVANCED_FACE('',(#2011),#1408,.F.);
#14747=ADVANCED_FACE('',(#2012),#972,.F.);
#14748=ADVANCED_FACE('',(#2013),#1409,.F.);
#14749=ADVANCED_FACE('',(#2014),#973,.F.);
#14750=ADVANCED_FACE('',(#2015),#1410,.F.);
#14751=ADVANCED_FACE('',(#2016),#974,.F.);
#14752=ADVANCED_FACE('',(#2017),#1411,.F.);
#14753=ADVANCED_FACE('',(#2018),#975,.F.);
#14754=ADVANCED_FACE('',(#2019),#1412,.F.);
#14755=ADVANCED_FACE('',(#2020),#976,.F.);
#14756=ADVANCED_FACE('',(#2021),#1413,.F.);
#14757=ADVANCED_FACE('',(#2022),#977,.F.);
#14758=ADVANCED_FACE('',(#2023),#1414,.F.);
#14759=ADVANCED_FACE('',(#2024),#978,.F.);
#14760=ADVANCED_FACE('',(#2025),#1415,.F.);
#14761=ADVANCED_FACE('',(#2026),#979,.F.);
#14762=ADVANCED_FACE('',(#2027),#1416,.F.);
#14763=ADVANCED_FACE('',(#2028),#980,.F.);
#14764=ADVANCED_FACE('',(#2029),#1417,.F.);
#14765=ADVANCED_FACE('',(#2030),#981,.F.);
#14766=ADVANCED_FACE('',(#2031),#1418,.F.);
#14767=ADVANCED_FACE('',(#2032),#982,.F.);
#14768=ADVANCED_FACE('',(#2033),#1419,.F.);
#14769=ADVANCED_FACE('',(#2034),#983,.F.);
#14770=ADVANCED_FACE('',(#2035),#1420,.F.);
#14771=ADVANCED_FACE('',(#2036),#984,.F.);
#14772=ADVANCED_FACE('',(#2037),#1421,.F.);
#14773=ADVANCED_FACE('',(#2038),#985,.F.);
#14774=ADVANCED_FACE('',(#2039),#1422,.T.);
#14775=ADVANCED_FACE('',(#2040),#986,.T.);
#14776=ADVANCED_FACE('',(#2041),#1423,.T.);
#14777=ADVANCED_FACE('',(#2042),#987,.T.);
#14778=ADVANCED_FACE('',(#2043),#1424,.T.);
#14779=ADVANCED_FACE('',(#2044),#988,.T.);
#14780=ADVANCED_FACE('',(#2045),#1425,.T.);
#14781=ADVANCED_FACE('',(#2046),#989,.T.);
#14782=ADVANCED_FACE('',(#2047,#1176,#1177,#1178,#1179,#1180,#1181,#1182,
#1183,#1184,#1185,#1186,#1187,#1188,#1189,#1190),#1426,.T.);
#14783=ADVANCED_FACE('',(#2048,#1191,#1192,#1193,#1194,#1195,#1196,#1197,
#1198,#1199,#1200,#1201,#1202,#1203,#1204,#1205),#1427,.F.);
#15088=CLOSED_SHELL('',(#14654,#14655,#14656,#14657,#14658,#14659,#14660,
#14661,#14662,#14663,#14664,#14665,#14666,#14667,#14668,#14669,#14670,#14671,
#14672,#14673,#14674,#14675,#14676,#14677,#14678,#14679,#14680,#14681,#14682,
#14683,#14684,#14685,#14686,#14687,#14688,#14689,#14690,#14691,#14692,#14693,
#14694,#14695,#14696,#14697,#14698,#14699,#14700,#14701,#14702,#14703,#14704,
#14705,#14706,#14707,#14708,#14709,#14710,#14711,#14712,#14713,#14714,#14715,
#14716,#14717,#14718,#14719,#14720,#14721,#14722,#14723,#14724,#14725,#14726,
#14727,#14728,#14729,#14730,#14731,#14732,#14733,#14734,#14735,#14736,#14737,
#14738,#14739,#14740,#14741,#14742,#14743,#14744,#14745,#14746,#14747,#14748,
#14749,#14750,#14751,#14752,#14753,#14754,#14755,#14756,#14757,#14758,#14759,
#14760,#14761,#14762,#14763,#14764,#14765,#14766,#14767,#14768,#14769,#14770,
#14771,#14772,#14773,#14774,#14775,#14776,#14777,#14778,#14779,#14780,#14781,
#14782,#14783));
#15816=AXIS2_PLACEMENT_3D('',#22246,#18352,#18353);
#15817=AXIS2_PLACEMENT_3D('',#22247,#18354,#18355);
#15818=AXIS2_PLACEMENT_3D('',#22256,#18360,#18361);
#15819=AXIS2_PLACEMENT_3D('',#22258,#18362,#18363);
#15820=AXIS2_PLACEMENT_3D('',#22261,#18365,#18366);
#15821=AXIS2_PLACEMENT_3D('',#22262,#18367,#18368);
#15822=AXIS2_PLACEMENT_3D('',#22268,#18372,#18373);
#15823=AXIS2_PLACEMENT_3D('',#22270,#18374,#18375);
#15824=AXIS2_PLACEMENT_3D('',#22273,#18377,#18378);
#15825=AXIS2_PLACEMENT_3D('',#22274,#18379,#18380);
#15826=AXIS2_PLACEMENT_3D('',#22280,#18384,#18385);
#15827=AXIS2_PLACEMENT_3D('',#22282,#18386,#18387);
#15828=AXIS2_PLACEMENT_3D('',#22285,#18389,#18390);
#15829=AXIS2_PLACEMENT_3D('',#22286,#18391,#18392);
#15830=AXIS2_PLACEMENT_3D('',#22292,#18396,#18397);
#15831=AXIS2_PLACEMENT_3D('',#22293,#18398,#18399);
#15832=AXIS2_PLACEMENT_3D('',#22294,#18400,#18401);
#15833=AXIS2_PLACEMENT_3D('',#22295,#18402,#18403);
#15834=AXIS2_PLACEMENT_3D('',#22304,#18408,#18409);
#15835=AXIS2_PLACEMENT_3D('',#22306,#18410,#18411);
#15836=AXIS2_PLACEMENT_3D('',#22309,#18413,#18414);
#15837=AXIS2_PLACEMENT_3D('',#22310,#18415,#18416);
#15838=AXIS2_PLACEMENT_3D('',#22316,#18420,#18421);
#15839=AXIS2_PLACEMENT_3D('',#22318,#18422,#18423);
#15840=AXIS2_PLACEMENT_3D('',#22321,#18425,#18426);
#15841=AXIS2_PLACEMENT_3D('',#22322,#18427,#18428);
#15842=AXIS2_PLACEMENT_3D('',#22328,#18432,#18433);
#15843=AXIS2_PLACEMENT_3D('',#22330,#18434,#18435);
#15844=AXIS2_PLACEMENT_3D('',#22333,#18437,#18438);
#15845=AXIS2_PLACEMENT_3D('',#22334,#18439,#18440);
#15846=AXIS2_PLACEMENT_3D('',#22340,#18444,#18445);
#15847=AXIS2_PLACEMENT_3D('',#22341,#18446,#18447);
#15848=AXIS2_PLACEMENT_3D('',#22342,#18448,#18449);
#15849=AXIS2_PLACEMENT_3D('',#22343,#18450,#18451);
#15850=AXIS2_PLACEMENT_3D('',#22352,#18456,#18457);
#15851=AXIS2_PLACEMENT_3D('',#22354,#18458,#18459);
#15852=AXIS2_PLACEMENT_3D('',#22357,#18461,#18462);
#15853=AXIS2_PLACEMENT_3D('',#22358,#18463,#18464);
#15854=AXIS2_PLACEMENT_3D('',#22364,#18468,#18469);
#15855=AXIS2_PLACEMENT_3D('',#22366,#18470,#18471);
#15856=AXIS2_PLACEMENT_3D('',#22369,#18473,#18474);
#15857=AXIS2_PLACEMENT_3D('',#22370,#18475,#18476);
#15858=AXIS2_PLACEMENT_3D('',#22376,#18480,#18481);
#15859=AXIS2_PLACEMENT_3D('',#22378,#18482,#18483);
#15860=AXIS2_PLACEMENT_3D('',#22381,#18485,#18486);
#15861=AXIS2_PLACEMENT_3D('',#22382,#18487,#18488);
#15862=AXIS2_PLACEMENT_3D('',#22388,#18492,#18493);
#15863=AXIS2_PLACEMENT_3D('',#22389,#18494,#18495);
#15864=AXIS2_PLACEMENT_3D('',#22390,#18496,#18497);
#15865=AXIS2_PLACEMENT_3D('',#22391,#18498,#18499);
#15866=AXIS2_PLACEMENT_3D('',#22400,#18504,#18505);
#15867=AXIS2_PLACEMENT_3D('',#22402,#18506,#18507);
#15868=AXIS2_PLACEMENT_3D('',#22405,#18509,#18510);
#15869=AXIS2_PLACEMENT_3D('',#22406,#18511,#18512);
#15870=AXIS2_PLACEMENT_3D('',#22412,#18516,#18517);
#15871=AXIS2_PLACEMENT_3D('',#22414,#18518,#18519);
#15872=AXIS2_PLACEMENT_3D('',#22417,#18521,#18522);
#15873=AXIS2_PLACEMENT_3D('',#22418,#18523,#18524);
#15874=AXIS2_PLACEMENT_3D('',#22424,#18528,#18529);
#15875=AXIS2_PLACEMENT_3D('',#22426,#18530,#18531);
#15876=AXIS2_PLACEMENT_3D('',#22429,#18533,#18534);
#15877=AXIS2_PLACEMENT_3D('',#22430,#18535,#18536);
#15878=AXIS2_PLACEMENT_3D('',#22436,#18540,#18541);
#15879=AXIS2_PLACEMENT_3D('',#22437,#18542,#18543);
#15880=AXIS2_PLACEMENT_3D('',#22438,#18544,#18545);
#15881=AXIS2_PLACEMENT_3D('',#22439,#18546,#18547);
#15882=AXIS2_PLACEMENT_3D('',#22448,#18552,#18553);
#15883=AXIS2_PLACEMENT_3D('',#22450,#18554,#18555);
#15884=AXIS2_PLACEMENT_3D('',#22453,#18557,#18558);
#15885=AXIS2_PLACEMENT_3D('',#22454,#18559,#18560);
#15886=AXIS2_PLACEMENT_3D('',#22460,#18564,#18565);
#15887=AXIS2_PLACEMENT_3D('',#22462,#18566,#18567);
#15888=AXIS2_PLACEMENT_3D('',#22465,#18569,#18570);
#15889=AXIS2_PLACEMENT_3D('',#22466,#18571,#18572);
#15890=AXIS2_PLACEMENT_3D('',#22472,#18576,#18577);
#15891=AXIS2_PLACEMENT_3D('',#22474,#18578,#18579);
#15892=AXIS2_PLACEMENT_3D('',#22477,#18581,#18582);
#15893=AXIS2_PLACEMENT_3D('',#22478,#18583,#18584);
#15894=AXIS2_PLACEMENT_3D('',#22484,#18588,#18589);
#15895=AXIS2_PLACEMENT_3D('',#22485,#18590,#18591);
#15896=AXIS2_PLACEMENT_3D('',#22486,#18592,#18593);
#15897=AXIS2_PLACEMENT_3D('',#22487,#18594,#18595);
#15898=AXIS2_PLACEMENT_3D('',#22496,#18600,#18601);
#15899=AXIS2_PLACEMENT_3D('',#22498,#18602,#18603);
#15900=AXIS2_PLACEMENT_3D('',#22501,#18605,#18606);
#15901=AXIS2_PLACEMENT_3D('',#22502,#18607,#18608);
#15902=AXIS2_PLACEMENT_3D('',#22508,#18612,#18613);
#15903=AXIS2_PLACEMENT_3D('',#22510,#18614,#18615);
#15904=AXIS2_PLACEMENT_3D('',#22513,#18617,#18618);
#15905=AXIS2_PLACEMENT_3D('',#22514,#18619,#18620);
#15906=AXIS2_PLACEMENT_3D('',#22520,#18624,#18625);
#15907=AXIS2_PLACEMENT_3D('',#22522,#18626,#18627);
#15908=AXIS2_PLACEMENT_3D('',#22525,#18629,#18630);
#15909=AXIS2_PLACEMENT_3D('',#22526,#18631,#18632);
#15910=AXIS2_PLACEMENT_3D('',#22532,#18636,#18637);
#15911=AXIS2_PLACEMENT_3D('',#22533,#18638,#18639);
#15912=AXIS2_PLACEMENT_3D('',#22534,#18640,#18641);
#15913=AXIS2_PLACEMENT_3D('',#22535,#18642,#18643);
#15914=AXIS2_PLACEMENT_3D('',#22544,#18648,#18649);
#15915=AXIS2_PLACEMENT_3D('',#22546,#18650,#18651);
#15916=AXIS2_PLACEMENT_3D('',#22549,#18653,#18654);
#15917=AXIS2_PLACEMENT_3D('',#22550,#18655,#18656);
#15918=AXIS2_PLACEMENT_3D('',#22556,#18660,#18661);
#15919=AXIS2_PLACEMENT_3D('',#22558,#18662,#18663);
#15920=AXIS2_PLACEMENT_3D('',#22561,#18665,#18666);
#15921=AXIS2_PLACEMENT_3D('',#22562,#18667,#18668);
#15922=AXIS2_PLACEMENT_3D('',#22568,#18672,#18673);
#15923=AXIS2_PLACEMENT_3D('',#22570,#18674,#18675);
#15924=AXIS2_PLACEMENT_3D('',#22573,#18677,#18678);
#15925=AXIS2_PLACEMENT_3D('',#22574,#18679,#18680);
#15926=AXIS2_PLACEMENT_3D('',#22580,#18684,#18685);
#15927=AXIS2_PLACEMENT_3D('',#22581,#18686,#18687);
#15928=AXIS2_PLACEMENT_3D('',#22582,#18688,#18689);
#15929=AXIS2_PLACEMENT_3D('',#22583,#18690,#18691);
#15930=AXIS2_PLACEMENT_3D('',#22592,#18696,#18697);
#15931=AXIS2_PLACEMENT_3D('',#22594,#18698,#18699);
#15932=AXIS2_PLACEMENT_3D('',#22597,#18701,#18702);
#15933=AXIS2_PLACEMENT_3D('',#22598,#18703,#18704);
#15934=AXIS2_PLACEMENT_3D('',#22604,#18708,#18709);
#15935=AXIS2_PLACEMENT_3D('',#22606,#18710,#18711);
#15936=AXIS2_PLACEMENT_3D('',#22609,#18713,#18714);
#15937=AXIS2_PLACEMENT_3D('',#22610,#18715,#18716);
#15938=AXIS2_PLACEMENT_3D('',#22616,#18720,#18721);
#15939=AXIS2_PLACEMENT_3D('',#22618,#18722,#18723);
#15940=AXIS2_PLACEMENT_3D('',#22621,#18725,#18726);
#15941=AXIS2_PLACEMENT_3D('',#22622,#18727,#18728);
#15942=AXIS2_PLACEMENT_3D('',#22628,#18732,#18733);
#15943=AXIS2_PLACEMENT_3D('',#22629,#18734,#18735);
#15944=AXIS2_PLACEMENT_3D('',#22630,#18736,#18737);
#15945=AXIS2_PLACEMENT_3D('',#22631,#18738,#18739);
#15946=AXIS2_PLACEMENT_3D('',#22640,#18744,#18745);
#15947=AXIS2_PLACEMENT_3D('',#22642,#18746,#18747);
#15948=AXIS2_PLACEMENT_3D('',#22645,#18749,#18750);
#15949=AXIS2_PLACEMENT_3D('',#22646,#18751,#18752);
#15950=AXIS2_PLACEMENT_3D('',#22652,#18756,#18757);
#15951=AXIS2_PLACEMENT_3D('',#22654,#18758,#18759);
#15952=AXIS2_PLACEMENT_3D('',#22657,#18761,#18762);
#15953=AXIS2_PLACEMENT_3D('',#22658,#18763,#18764);
#15954=AXIS2_PLACEMENT_3D('',#22664,#18768,#18769);
#15955=AXIS2_PLACEMENT_3D('',#22666,#18770,#18771);
#15956=AXIS2_PLACEMENT_3D('',#22669,#18773,#18774);
#15957=AXIS2_PLACEMENT_3D('',#22670,#18775,#18776);
#15958=AXIS2_PLACEMENT_3D('',#22676,#18780,#18781);
#15959=AXIS2_PLACEMENT_3D('',#22677,#18782,#18783);
#15960=AXIS2_PLACEMENT_3D('',#22678,#18784,#18785);
#15961=AXIS2_PLACEMENT_3D('',#22679,#18786,#18787);
#15962=AXIS2_PLACEMENT_3D('',#22688,#18792,#18793);
#15963=AXIS2_PLACEMENT_3D('',#22690,#18794,#18795);
#15964=AXIS2_PLACEMENT_3D('',#22693,#18797,#18798);
#15965=AXIS2_PLACEMENT_3D('',#22694,#18799,#18800);
#15966=AXIS2_PLACEMENT_3D('',#22700,#18804,#18805);
#15967=AXIS2_PLACEMENT_3D('',#22702,#18806,#18807);
#15968=AXIS2_PLACEMENT_3D('',#22705,#18809,#18810);
#15969=AXIS2_PLACEMENT_3D('',#22706,#18811,#18812);
#15970=AXIS2_PLACEMENT_3D('',#22712,#18816,#18817);
#15971=AXIS2_PLACEMENT_3D('',#22714,#18818,#18819);
#15972=AXIS2_PLACEMENT_3D('',#22717,#18821,#18822);
#15973=AXIS2_PLACEMENT_3D('',#22718,#18823,#18824);
#15974=AXIS2_PLACEMENT_3D('',#22724,#18828,#18829);
#15975=AXIS2_PLACEMENT_3D('',#22725,#18830,#18831);
#15976=AXIS2_PLACEMENT_3D('',#22726,#18832,#18833);
#15977=AXIS2_PLACEMENT_3D('',#22727,#18834,#18835);
#15978=AXIS2_PLACEMENT_3D('',#22736,#18840,#18841);
#15979=AXIS2_PLACEMENT_3D('',#22738,#18842,#18843);
#15980=AXIS2_PLACEMENT_3D('',#22741,#18845,#18846);
#15981=AXIS2_PLACEMENT_3D('',#22742,#18847,#18848);
#15982=AXIS2_PLACEMENT_3D('',#22748,#18852,#18853);
#15983=AXIS2_PLACEMENT_3D('',#22750,#18854,#18855);
#15984=AXIS2_PLACEMENT_3D('',#22753,#18857,#18858);
#15985=AXIS2_PLACEMENT_3D('',#22754,#18859,#18860);
#15986=AXIS2_PLACEMENT_3D('',#22760,#18864,#18865);
#15987=AXIS2_PLACEMENT_3D('',#22762,#18866,#18867);
#15988=AXIS2_PLACEMENT_3D('',#22765,#18869,#18870);
#15989=AXIS2_PLACEMENT_3D('',#22766,#18871,#18872);
#15990=AXIS2_PLACEMENT_3D('',#22772,#18876,#18877);
#15991=AXIS2_PLACEMENT_3D('',#22773,#18878,#18879);
#15992=AXIS2_PLACEMENT_3D('',#22774,#18880,#18881);
#15993=AXIS2_PLACEMENT_3D('',#22775,#18882,#18883);
#15994=AXIS2_PLACEMENT_3D('',#22784,#18888,#18889);
#15995=AXIS2_PLACEMENT_3D('',#22786,#18890,#18891);
#15996=AXIS2_PLACEMENT_3D('',#22789,#18893,#18894);
#15997=AXIS2_PLACEMENT_3D('',#22790,#18895,#18896);
#15998=AXIS2_PLACEMENT_3D('',#22796,#18900,#18901);
#15999=AXIS2_PLACEMENT_3D('',#22798,#18902,#18903);
#16000=AXIS2_PLACEMENT_3D('',#22801,#18905,#18906);
#16001=AXIS2_PLACEMENT_3D('',#22802,#18907,#18908);
#16002=AXIS2_PLACEMENT_3D('',#22808,#18912,#18913);
#16003=AXIS2_PLACEMENT_3D('',#22810,#18914,#18915);
#16004=AXIS2_PLACEMENT_3D('',#22813,#18917,#18918);
#16005=AXIS2_PLACEMENT_3D('',#22814,#18919,#18920);
#16006=AXIS2_PLACEMENT_3D('',#22820,#18924,#18925);
#16007=AXIS2_PLACEMENT_3D('',#22821,#18926,#18927);
#16008=AXIS2_PLACEMENT_3D('',#22822,#18928,#18929);
#16009=AXIS2_PLACEMENT_3D('',#22823,#18930,#18931);
#16010=AXIS2_PLACEMENT_3D('',#22832,#18936,#18937);
#16011=AXIS2_PLACEMENT_3D('',#22834,#18938,#18939);
#16012=AXIS2_PLACEMENT_3D('',#22837,#18941,#18942);
#16013=AXIS2_PLACEMENT_3D('',#22838,#18943,#18944);
#16014=AXIS2_PLACEMENT_3D('',#22844,#18948,#18949);
#16015=AXIS2_PLACEMENT_3D('',#22846,#18950,#18951);
#16016=AXIS2_PLACEMENT_3D('',#22849,#18953,#18954);
#16017=AXIS2_PLACEMENT_3D('',#22850,#18955,#18956);
#16018=AXIS2_PLACEMENT_3D('',#22856,#18960,#18961);
#16019=AXIS2_PLACEMENT_3D('',#22858,#18962,#18963);
#16020=AXIS2_PLACEMENT_3D('',#22861,#18965,#18966);
#16021=AXIS2_PLACEMENT_3D('',#22862,#18967,#18968);
#16022=AXIS2_PLACEMENT_3D('',#22868,#18972,#18973);
#16023=AXIS2_PLACEMENT_3D('',#22869,#18974,#18975);
#16024=AXIS2_PLACEMENT_3D('',#22870,#18976,#18977);
#16025=AXIS2_PLACEMENT_3D('',#22871,#18978,#18979);
#16026=AXIS2_PLACEMENT_3D('',#22880,#18984,#18985);
#16027=AXIS2_PLACEMENT_3D('',#22882,#18986,#18987);
#16028=AXIS2_PLACEMENT_3D('',#22885,#18989,#18990);
#16029=AXIS2_PLACEMENT_3D('',#22886,#18991,#18992);
#16030=AXIS2_PLACEMENT_3D('',#22892,#18996,#18997);
#16031=AXIS2_PLACEMENT_3D('',#22894,#18998,#18999);
#16032=AXIS2_PLACEMENT_3D('',#22897,#19001,#19002);
#16033=AXIS2_PLACEMENT_3D('',#22898,#19003,#19004);
#16034=AXIS2_PLACEMENT_3D('',#22904,#19008,#19009);
#16035=AXIS2_PLACEMENT_3D('',#22906,#19010,#19011);
#16036=AXIS2_PLACEMENT_3D('',#22909,#19013,#19014);
#16037=AXIS2_PLACEMENT_3D('',#22910,#19015,#19016);
#16038=AXIS2_PLACEMENT_3D('',#22916,#19020,#19021);
#16039=AXIS2_PLACEMENT_3D('',#22917,#19022,#19023);
#16040=AXIS2_PLACEMENT_3D('',#22918,#19024,#19025);
#16041=AXIS2_PLACEMENT_3D('',#22919,#19026,#19027);
#16042=AXIS2_PLACEMENT_3D('',#22928,#19032,#19033);
#16043=AXIS2_PLACEMENT_3D('',#22930,#19034,#19035);
#16044=AXIS2_PLACEMENT_3D('',#22933,#19037,#19038);
#16045=AXIS2_PLACEMENT_3D('',#22934,#19039,#19040);
#16046=AXIS2_PLACEMENT_3D('',#22940,#19044,#19045);
#16047=AXIS2_PLACEMENT_3D('',#22942,#19046,#19047);
#16048=AXIS2_PLACEMENT_3D('',#22945,#19049,#19050);
#16049=AXIS2_PLACEMENT_3D('',#22946,#19051,#19052);
#16050=AXIS2_PLACEMENT_3D('',#22952,#19056,#19057);
#16051=AXIS2_PLACEMENT_3D('',#22954,#19058,#19059);
#16052=AXIS2_PLACEMENT_3D('',#22957,#19061,#19062);
#16053=AXIS2_PLACEMENT_3D('',#22958,#19063,#19064);
#16054=AXIS2_PLACEMENT_3D('',#22964,#19068,#19069);
#16055=AXIS2_PLACEMENT_3D('',#22965,#19070,#19071);
#16056=AXIS2_PLACEMENT_3D('',#22966,#19072,#19073);
#16057=AXIS2_PLACEMENT_3D('',#22967,#19074,#19075);
#16058=AXIS2_PLACEMENT_3D('',#22976,#19080,#19081);
#16059=AXIS2_PLACEMENT_3D('',#22978,#19082,#19083);
#16060=AXIS2_PLACEMENT_3D('',#22980,#19084,#19085);
#16061=AXIS2_PLACEMENT_3D('',#22982,#19087,#19088);
#16062=AXIS2_PLACEMENT_3D('',#22988,#19092,#19093);
#16063=AXIS2_PLACEMENT_3D('',#22990,#19094,#19095);
#16064=AXIS2_PLACEMENT_3D('',#22992,#19096,#19097);
#16065=AXIS2_PLACEMENT_3D('',#22994,#19099,#19100);
#16066=AXIS2_PLACEMENT_3D('',#23000,#19104,#19105);
#16067=AXIS2_PLACEMENT_3D('',#23002,#19106,#19107);
#16068=AXIS2_PLACEMENT_3D('',#23004,#19108,#19109);
#16069=AXIS2_PLACEMENT_3D('',#23006,#19111,#19112);
#16070=AXIS2_PLACEMENT_3D('',#23012,#19116,#19117);
#16071=AXIS2_PLACEMENT_3D('',#23013,#19118,#19119);
#16072=AXIS2_PLACEMENT_3D('',#23014,#19120,#19121);
#16073=AXIS2_PLACEMENT_3D('',#23015,#19122,#19123);
#16074=AXIS2_PLACEMENT_3D('',#23016,#19124,#19125);
#18352=DIRECTION('axis',(0.,0.,1.));
#18353=DIRECTION('refdir',(1.,0.,0.));
#18354=DIRECTION('center_axis',(-1.,0.,0.));
#18355=DIRECTION('ref_axis',(0.,-1.,0.));
#18356=DIRECTION('',(0.,-1.,0.));
#18357=DIRECTION('',(0.,0.,1.));
#18358=DIRECTION('',(0.,1.,0.));
#18359=DIRECTION('',(0.,0.,1.));
#18360=DIRECTION('center_axis',(0.,0.,1.));
#18361=DIRECTION('ref_axis',(-8.88178419700065E-14,1.,0.));
#18362=DIRECTION('center_axis',(0.,0.,1.));
#18363=DIRECTION('ref_axis',(-8.88178419700065E-14,1.,0.));
#18364=DIRECTION('',(0.,0.,1.));
#18365=DIRECTION('center_axis',(0.,0.,-1.));
#18366=DIRECTION('ref_axis',(-8.88178419700065E-14,1.,0.));
#18367=DIRECTION('center_axis',(0.,1.,0.));
#18368=DIRECTION('ref_axis',(-1.,0.,0.));
#18369=DIRECTION('',(-1.,0.,0.));
#18370=DIRECTION('',(0.,0.,1.));
#18371=DIRECTION('',(1.,0.,0.));
#18372=DIRECTION('center_axis',(0.,0.,1.));
#18373=DIRECTION('ref_axis',(1.,-1.33226762955033E-13,0.));
#18374=DIRECTION('center_axis',(0.,0.,1.));
#18375=DIRECTION('ref_axis',(1.,-1.33226762955033E-13,0.));
#18376=DIRECTION('',(0.,0.,1.));
#18377=DIRECTION('center_axis',(0.,0.,-1.));
#18378=DIRECTION('ref_axis',(1.,-1.33226762955033E-13,0.));
#18379=DIRECTION('center_axis',(1.,0.,0.));
#18380=DIRECTION('ref_axis',(0.,1.,0.));
#18381=DIRECTION('',(0.,1.,0.));
#18382=DIRECTION('',(0.,0.,1.));
#18383=DIRECTION('',(0.,-1.,0.));
#18384=DIRECTION('center_axis',(0.,0.,1.));
#18385=DIRECTION('ref_axis',(-8.88178419700248E-14,-1.,0.));
#18386=DIRECTION('center_axis',(0.,0.,1.));
#18387=DIRECTION('ref_axis',(-8.88178419700248E-14,-1.,0.));
#18388=DIRECTION('',(0.,0.,1.));
#18389=DIRECTION('center_axis',(0.,0.,-1.));
#18390=DIRECTION('ref_axis',(-8.88178419700248E-14,-1.,0.));
#18391=DIRECTION('center_axis',(0.,-1.,0.));
#18392=DIRECTION('ref_axis',(1.,0.,0.));
#18393=DIRECTION('',(1.,0.,0.));
#18394=DIRECTION('',(0.,0.,1.));
#18395=DIRECTION('',(-1.,0.,0.));
#18396=DIRECTION('center_axis',(0.,0.,1.));
#18397=DIRECTION('ref_axis',(-1.,-6.66133814775049E-14,0.));
#18398=DIRECTION('center_axis',(0.,0.,1.));
#18399=DIRECTION('ref_axis',(-1.,-6.66133814775049E-14,0.));
#18400=DIRECTION('center_axis',(0.,0.,-1.));
#18401=DIRECTION('ref_axis',(-1.,-6.66133814775049E-14,0.));
#18402=DIRECTION('center_axis',(-1.,0.,0.));
#18403=DIRECTION('ref_axis',(0.,-1.,0.));
#18404=DIRECTION('',(0.,-1.,0.));
#18405=DIRECTION('',(0.,0.,1.));
#18406=DIRECTION('',(0.,1.,0.));
#18407=DIRECTION('',(0.,0.,1.));
#18408=DIRECTION('center_axis',(0.,0.,1.));
#18409=DIRECTION('ref_axis',(1.11022302462517E-14,1.,0.));
#18410=DIRECTION('center_axis',(0.,0.,1.));
#18411=DIRECTION('ref_axis',(1.11022302462517E-14,1.,0.));
#18412=DIRECTION('',(0.,0.,1.));
#18413=DIRECTION('center_axis',(0.,0.,-1.));
#18414=DIRECTION('ref_axis',(1.11022302462517E-14,1.,0.));
#18415=DIRECTION('center_axis',(0.,1.,0.));
#18416=DIRECTION('ref_axis',(-1.,0.,0.));
#18417=DIRECTION('',(-1.,0.,0.));
#18418=DIRECTION('',(0.,0.,1.));
#18419=DIRECTION('',(1.,0.,0.));
#18420=DIRECTION('center_axis',(0.,0.,1.));
#18421=DIRECTION('ref_axis',(1.,-1.11022302462516E-14,0.));
#18422=DIRECTION('center_axis',(0.,0.,1.));
#18423=DIRECTION('ref_axis',(1.,-1.11022302462516E-14,0.));
#18424=DIRECTION('',(0.,0.,1.));
#18425=DIRECTION('center_axis',(0.,0.,-1.));
#18426=DIRECTION('ref_axis',(1.,-1.11022302462516E-14,0.));
#18427=DIRECTION('center_axis',(1.,0.,0.));
#18428=DIRECTION('ref_axis',(0.,1.,0.));
#18429=DIRECTION('',(0.,1.,0.));
#18430=DIRECTION('',(0.,0.,1.));
#18431=DIRECTION('',(0.,-1.,0.));
#18432=DIRECTION('center_axis',(0.,0.,1.));
#18433=DIRECTION('ref_axis',(2.22044604925034E-14,-1.,0.));
#18434=DIRECTION('center_axis',(0.,0.,1.));
#18435=DIRECTION('ref_axis',(2.22044604925034E-14,-1.,0.));
#18436=DIRECTION('',(0.,0.,1.));
#18437=DIRECTION('center_axis',(0.,0.,-1.));
#18438=DIRECTION('ref_axis',(2.22044604925034E-14,-1.,0.));
#18439=DIRECTION('center_axis',(0.,-1.,0.));
#18440=DIRECTION('ref_axis',(1.,0.,0.));
#18441=DIRECTION('',(1.,0.,0.));
#18442=DIRECTION('',(0.,0.,1.));
#18443=DIRECTION('',(-1.,0.,0.));
#18444=DIRECTION('center_axis',(0.,0.,1.));
#18445=DIRECTION('ref_axis',(-1.,5.55111512312584E-15,0.));
#18446=DIRECTION('center_axis',(0.,0.,1.));
#18447=DIRECTION('ref_axis',(-1.,5.55111512312584E-15,0.));
#18448=DIRECTION('center_axis',(0.,0.,-1.));
#18449=DIRECTION('ref_axis',(-1.,5.55111512312584E-15,0.));
#18450=DIRECTION('center_axis',(-1.,0.,0.));
#18451=DIRECTION('ref_axis',(0.,-1.,0.));
#18452=DIRECTION('',(0.,-1.,0.));
#18453=DIRECTION('',(0.,0.,1.));
#18454=DIRECTION('',(0.,1.,0.));
#18455=DIRECTION('',(0.,0.,1.));
#18456=DIRECTION('center_axis',(0.,0.,1.));
#18457=DIRECTION('ref_axis',(-2.96059473233373E-14,1.,0.));
#18458=DIRECTION('center_axis',(0.,0.,1.));
#18459=DIRECTION('ref_axis',(-2.96059473233373E-14,1.,0.));
#18460=DIRECTION('',(0.,0.,1.));
#18461=DIRECTION('center_axis',(0.,0.,-1.));
#18462=DIRECTION('ref_axis',(-2.96059473233373E-14,1.,0.));
#18463=DIRECTION('center_axis',(0.,1.,0.));
#18464=DIRECTION('ref_axis',(-1.,0.,0.));
#18465=DIRECTION('',(-1.,0.,0.));
#18466=DIRECTION('',(0.,0.,1.));
#18467=DIRECTION('',(1.,0.,0.));
#18468=DIRECTION('center_axis',(0.,0.,1.));
#18469=DIRECTION('ref_axis',(1.,0.,0.));
#18470=DIRECTION('center_axis',(0.,0.,1.));
#18471=DIRECTION('ref_axis',(1.,0.,0.));
#18472=DIRECTION('',(0.,0.,1.));
#18473=DIRECTION('center_axis',(0.,0.,-1.));
#18474=DIRECTION('ref_axis',(1.,0.,0.));
#18475=DIRECTION('center_axis',(1.,0.,0.));
#18476=DIRECTION('ref_axis',(0.,1.,0.));
#18477=DIRECTION('',(0.,1.,0.));
#18478=DIRECTION('',(0.,0.,1.));
#18479=DIRECTION('',(0.,-1.,0.));
#18480=DIRECTION('center_axis',(0.,0.,1.));
#18481=DIRECTION('ref_axis',(2.96059473233373E-14,-1.,0.));
#18482=DIRECTION('center_axis',(0.,0.,1.));
#18483=DIRECTION('ref_axis',(2.96059473233373E-14,-1.,0.));
#18484=DIRECTION('',(0.,0.,1.));
#18485=DIRECTION('center_axis',(0.,0.,-1.));
#18486=DIRECTION('ref_axis',(2.96059473233373E-14,-1.,0.));
#18487=DIRECTION('center_axis',(0.,-1.,0.));
#18488=DIRECTION('ref_axis',(1.,0.,0.));
#18489=DIRECTION('',(1.,0.,0.));
#18490=DIRECTION('',(0.,0.,1.));
#18491=DIRECTION('',(-1.,0.,0.));
#18492=DIRECTION('center_axis',(0.,0.,1.));
#18493=DIRECTION('ref_axis',(-1.,-7.40148683083432E-15,0.));
#18494=DIRECTION('center_axis',(0.,0.,1.));
#18495=DIRECTION('ref_axis',(-1.,-7.40148683083432E-15,0.));
#18496=DIRECTION('center_axis',(0.,0.,-1.));
#18497=DIRECTION('ref_axis',(-1.,-7.40148683083432E-15,0.));
#18498=DIRECTION('center_axis',(-1.,0.,0.));
#18499=DIRECTION('ref_axis',(0.,-1.,0.));
#18500=DIRECTION('',(0.,-1.,0.));
#18501=DIRECTION('',(0.,0.,1.));
#18502=DIRECTION('',(0.,1.,0.));
#18503=DIRECTION('',(0.,0.,1.));
#18504=DIRECTION('center_axis',(0.,0.,1.));
#18505=DIRECTION('ref_axis',(-2.96059473233373E-14,1.,0.));
#18506=DIRECTION('center_axis',(0.,0.,1.));
#18507=DIRECTION('ref_axis',(-2.96059473233373E-14,1.,0.));
#18508=DIRECTION('',(0.,0.,1.));
#18509=DIRECTION('center_axis',(0.,0.,-1.));
#18510=DIRECTION('ref_axis',(-2.96059473233373E-14,1.,0.));
#18511=DIRECTION('center_axis',(0.,1.,0.));
#18512=DIRECTION('ref_axis',(-1.,0.,0.));
#18513=DIRECTION('',(-1.,0.,0.));
#18514=DIRECTION('',(0.,0.,1.));
#18515=DIRECTION('',(1.,0.,0.));
#18516=DIRECTION('center_axis',(0.,0.,1.));
#18517=DIRECTION('ref_axis',(1.,0.,0.));
#18518=DIRECTION('center_axis',(0.,0.,1.));
#18519=DIRECTION('ref_axis',(1.,0.,0.));
#18520=DIRECTION('',(0.,0.,1.));
#18521=DIRECTION('center_axis',(0.,0.,-1.));
#18522=DIRECTION('ref_axis',(1.,0.,0.));
#18523=DIRECTION('center_axis',(1.,0.,0.));
#18524=DIRECTION('ref_axis',(0.,1.,0.));
#18525=DIRECTION('',(0.,1.,0.));
#18526=DIRECTION('',(0.,0.,1.));
#18527=DIRECTION('',(0.,-1.,0.));
#18528=DIRECTION('center_axis',(0.,0.,1.));
#18529=DIRECTION('ref_axis',(2.96059473233373E-14,-1.,0.));
#18530=DIRECTION('center_axis',(0.,0.,1.));
#18531=DIRECTION('ref_axis',(2.96059473233373E-14,-1.,0.));
#18532=DIRECTION('',(0.,0.,1.));
#18533=DIRECTION('center_axis',(0.,0.,-1.));
#18534=DIRECTION('ref_axis',(2.96059473233373E-14,-1.,0.));
#18535=DIRECTION('center_axis',(0.,-1.,0.));
#18536=DIRECTION('ref_axis',(1.,0.,0.));
#18537=DIRECTION('',(1.,0.,0.));
#18538=DIRECTION('',(0.,0.,1.));
#18539=DIRECTION('',(-1.,0.,0.));
#18540=DIRECTION('center_axis',(0.,0.,1.));
#18541=DIRECTION('ref_axis',(-1.,-7.40148683083432E-15,0.));
#18542=DIRECTION('center_axis',(0.,0.,1.));
#18543=DIRECTION('ref_axis',(-1.,-7.40148683083432E-15,0.));
#18544=DIRECTION('center_axis',(0.,0.,-1.));
#18545=DIRECTION('ref_axis',(-1.,-7.40148683083432E-15,0.));
#18546=DIRECTION('center_axis',(-1.,0.,0.));
#18547=DIRECTION('ref_axis',(0.,-1.,0.));
#18548=DIRECTION('',(0.,-1.,0.));
#18549=DIRECTION('',(0.,0.,1.));
#18550=DIRECTION('',(0.,1.,0.));
#18551=DIRECTION('',(0.,0.,1.));
#18552=DIRECTION('center_axis',(0.,0.,1.));
#18553=DIRECTION('ref_axis',(0.,1.,0.));
#18554=DIRECTION('center_axis',(0.,0.,1.));
#18555=DIRECTION('ref_axis',(0.,1.,0.));
#18556=DIRECTION('',(0.,0.,1.));
#18557=DIRECTION('center_axis',(0.,0.,-1.));
#18558=DIRECTION('ref_axis',(0.,1.,0.));
#18559=DIRECTION('center_axis',(0.,1.,0.));
#18560=DIRECTION('ref_axis',(-1.,0.,0.));
#18561=DIRECTION('',(-1.,0.,0.));
#18562=DIRECTION('',(0.,0.,1.));
#18563=DIRECTION('',(1.,0.,0.));
#18564=DIRECTION('center_axis',(0.,0.,1.));
#18565=DIRECTION('ref_axis',(1.,-2.96059473233381E-14,0.));
#18566=DIRECTION('center_axis',(0.,0.,1.));
#18567=DIRECTION('ref_axis',(1.,-2.96059473233381E-14,0.));
#18568=DIRECTION('',(0.,0.,1.));
#18569=DIRECTION('center_axis',(0.,0.,-1.));
#18570=DIRECTION('ref_axis',(1.,-2.96059473233381E-14,0.));
#18571=DIRECTION('center_axis',(1.,0.,0.));
#18572=DIRECTION('ref_axis',(0.,1.,0.));
#18573=DIRECTION('',(0.,1.,0.));
#18574=DIRECTION('',(0.,0.,1.));
#18575=DIRECTION('',(0.,-1.,0.));
#18576=DIRECTION('center_axis',(0.,0.,1.));
#18577=DIRECTION('ref_axis',(0.,-1.,0.));
#18578=DIRECTION('center_axis',(0.,0.,1.));
#18579=DIRECTION('ref_axis',(0.,-1.,0.));
#18580=DIRECTION('',(0.,0.,1.));
#18581=DIRECTION('center_axis',(0.,0.,-1.));
#18582=DIRECTION('ref_axis',(0.,-1.,0.));
#18583=DIRECTION('center_axis',(0.,-1.,0.));
#18584=DIRECTION('ref_axis',(1.,0.,0.));
#18585=DIRECTION('',(1.,0.,0.));
#18586=DIRECTION('',(0.,0.,1.));
#18587=DIRECTION('',(-1.,0.,0.));
#18588=DIRECTION('center_axis',(0.,0.,1.));
#18589=DIRECTION('ref_axis',(-1.,2.22044604925036E-14,0.));
#18590=DIRECTION('center_axis',(0.,0.,1.));
#18591=DIRECTION('ref_axis',(-1.,2.22044604925036E-14,0.));
#18592=DIRECTION('center_axis',(0.,0.,-1.));
#18593=DIRECTION('ref_axis',(-1.,2.22044604925036E-14,0.));
#18594=DIRECTION('center_axis',(-1.,0.,0.));
#18595=DIRECTION('ref_axis',(0.,-1.,0.));
#18596=DIRECTION('',(0.,-1.,0.));
#18597=DIRECTION('',(0.,0.,1.));
#18598=DIRECTION('',(0.,1.,0.));
#18599=DIRECTION('',(0.,0.,1.));
#18600=DIRECTION('center_axis',(0.,0.,1.));
#18601=DIRECTION('ref_axis',(0.,1.,0.));
#18602=DIRECTION('center_axis',(0.,0.,1.));
#18603=DIRECTION('ref_axis',(0.,1.,0.));
#18604=DIRECTION('',(0.,0.,1.));
#18605=DIRECTION('center_axis',(0.,0.,-1.));
#18606=DIRECTION('ref_axis',(0.,1.,0.));
#18607=DIRECTION('center_axis',(0.,1.,0.));
#18608=DIRECTION('ref_axis',(-1.,0.,0.));
#18609=DIRECTION('',(-1.,0.,0.));
#18610=DIRECTION('',(0.,0.,1.));
#18611=DIRECTION('',(1.,0.,0.));
#18612=DIRECTION('center_axis',(0.,0.,1.));
#18613=DIRECTION('ref_axis',(1.,-2.96059473233381E-14,0.));
#18614=DIRECTION('center_axis',(0.,0.,1.));
#18615=DIRECTION('ref_axis',(1.,-2.96059473233381E-14,0.));
#18616=DIRECTION('',(0.,0.,1.));
#18617=DIRECTION('center_axis',(0.,0.,-1.));
#18618=DIRECTION('ref_axis',(1.,-2.96059473233381E-14,0.));
#18619=DIRECTION('center_axis',(1.,0.,0.));
#18620=DIRECTION('ref_axis',(0.,1.,0.));
#18621=DIRECTION('',(0.,1.,0.));
#18622=DIRECTION('',(0.,0.,1.));
#18623=DIRECTION('',(0.,-1.,0.));
#18624=DIRECTION('center_axis',(0.,0.,1.));
#18625=DIRECTION('ref_axis',(0.,-1.,0.));
#18626=DIRECTION('center_axis',(0.,0.,1.));
#18627=DIRECTION('ref_axis',(0.,-1.,0.));
#18628=DIRECTION('',(0.,0.,1.));
#18629=DIRECTION('center_axis',(0.,0.,-1.));
#18630=DIRECTION('ref_axis',(0.,-1.,0.));
#18631=DIRECTION('center_axis',(0.,-1.,0.));
#18632=DIRECTION('ref_axis',(1.,0.,0.));
#18633=DIRECTION('',(1.,0.,0.));
#18634=DIRECTION('',(0.,0.,1.));
#18635=DIRECTION('',(-1.,0.,0.));
#18636=DIRECTION('center_axis',(0.,0.,1.));
#18637=DIRECTION('ref_axis',(-1.,2.22044604925036E-14,0.));
#18638=DIRECTION('center_axis',(0.,0.,1.));
#18639=DIRECTION('ref_axis',(-1.,2.22044604925036E-14,0.));
#18640=DIRECTION('center_axis',(0.,0.,-1.));
#18641=DIRECTION('ref_axis',(-1.,2.22044604925036E-14,0.));
#18642=DIRECTION('center_axis',(-1.,0.,0.));
#18643=DIRECTION('ref_axis',(0.,-1.,0.));
#18644=DIRECTION('',(0.,-1.,0.));
#18645=DIRECTION('',(0.,0.,1.));
#18646=DIRECTION('',(0.,1.,0.));
#18647=DIRECTION('',(0.,0.,1.));
#18648=DIRECTION('center_axis',(0.,0.,1.));
#18649=DIRECTION('ref_axis',(0.,1.,0.));
#18650=DIRECTION('center_axis',(0.,0.,1.));
#18651=DIRECTION('ref_axis',(0.,1.,0.));
#18652=DIRECTION('',(0.,0.,1.));
#18653=DIRECTION('center_axis',(0.,0.,-1.));
#18654=DIRECTION('ref_axis',(0.,1.,0.));
#18655=DIRECTION('center_axis',(0.,1.,0.));
#18656=DIRECTION('ref_axis',(-1.,0.,0.));
#18657=DIRECTION('',(-1.,0.,0.));
#18658=DIRECTION('',(0.,0.,1.));
#18659=DIRECTION('',(1.,0.,0.));
#18660=DIRECTION('center_axis',(0.,0.,1.));
#18661=DIRECTION('ref_axis',(1.,-2.96059473233381E-14,0.));
#18662=DIRECTION('center_axis',(0.,0.,1.));
#18663=DIRECTION('ref_axis',(1.,-2.96059473233381E-14,0.));
#18664=DIRECTION('',(0.,0.,1.));
#18665=DIRECTION('center_axis',(0.,0.,-1.));
#18666=DIRECTION('ref_axis',(1.,-2.96059473233381E-14,0.));
#18667=DIRECTION('center_axis',(1.,0.,0.));
#18668=DIRECTION('ref_axis',(0.,1.,0.));
#18669=DIRECTION('',(0.,1.,0.));
#18670=DIRECTION('',(0.,0.,1.));
#18671=DIRECTION('',(0.,-1.,0.));
#18672=DIRECTION('center_axis',(0.,0.,1.));
#18673=DIRECTION('ref_axis',(0.,-1.,0.));
#18674=DIRECTION('center_axis',(0.,0.,1.));
#18675=DIRECTION('ref_axis',(0.,-1.,0.));
#18676=DIRECTION('',(0.,0.,1.));
#18677=DIRECTION('center_axis',(0.,0.,-1.));
#18678=DIRECTION('ref_axis',(0.,-1.,0.));
#18679=DIRECTION('center_axis',(0.,-1.,0.));
#18680=DIRECTION('ref_axis',(1.,0.,0.));
#18681=DIRECTION('',(1.,0.,0.));
#18682=DIRECTION('',(0.,0.,1.));
#18683=DIRECTION('',(-1.,0.,0.));
#18684=DIRECTION('center_axis',(0.,0.,1.));
#18685=DIRECTION('ref_axis',(-1.,2.22044604925036E-14,0.));
#18686=DIRECTION('center_axis',(0.,0.,1.));
#18687=DIRECTION('ref_axis',(-1.,2.22044604925036E-14,0.));
#18688=DIRECTION('center_axis',(0.,0.,-1.));
#18689=DIRECTION('ref_axis',(-1.,2.22044604925036E-14,0.));
#18690=DIRECTION('center_axis',(-1.,0.,0.));
#18691=DIRECTION('ref_axis',(0.,-1.,0.));
#18692=DIRECTION('',(0.,-1.,0.));
#18693=DIRECTION('',(0.,0.,1.));
#18694=DIRECTION('',(0.,1.,0.));
#18695=DIRECTION('',(0.,0.,1.));
#18696=DIRECTION('center_axis',(0.,0.,1.));
#18697=DIRECTION('ref_axis',(0.,1.,0.));
#18698=DIRECTION('center_axis',(0.,0.,1.));
#18699=DIRECTION('ref_axis',(0.,1.,0.));
#18700=DIRECTION('',(0.,0.,1.));
#18701=DIRECTION('center_axis',(0.,0.,-1.));
#18702=DIRECTION('ref_axis',(0.,1.,0.));
#18703=DIRECTION('center_axis',(0.,1.,0.));
#18704=DIRECTION('ref_axis',(-1.,0.,0.));
#18705=DIRECTION('',(-1.,0.,0.));
#18706=DIRECTION('',(0.,0.,1.));
#18707=DIRECTION('',(1.,0.,0.));
#18708=DIRECTION('center_axis',(0.,0.,1.));
#18709=DIRECTION('ref_axis',(1.,-1.48029736616686E-14,0.));
#18710=DIRECTION('center_axis',(0.,0.,1.));
#18711=DIRECTION('ref_axis',(1.,-1.48029736616686E-14,0.));
#18712=DIRECTION('',(0.,0.,1.));
#18713=DIRECTION('center_axis',(0.,0.,-1.));
#18714=DIRECTION('ref_axis',(1.,-1.48029736616686E-14,0.));
#18715=DIRECTION('center_axis',(1.,0.,0.));
#18716=DIRECTION('ref_axis',(0.,1.,0.));
#18717=DIRECTION('',(0.,1.,0.));
#18718=DIRECTION('',(0.,0.,1.));
#18719=DIRECTION('',(0.,-1.,0.));
#18720=DIRECTION('center_axis',(0.,0.,1.));
#18721=DIRECTION('ref_axis',(1.48029736616688E-14,-1.,0.));
#18722=DIRECTION('center_axis',(0.,0.,1.));
#18723=DIRECTION('ref_axis',(1.48029736616688E-14,-1.,0.));
#18724=DIRECTION('',(0.,0.,1.));
#18725=DIRECTION('center_axis',(0.,0.,-1.));
#18726=DIRECTION('ref_axis',(1.48029736616688E-14,-1.,0.));
#18727=DIRECTION('center_axis',(0.,-1.,0.));
#18728=DIRECTION('ref_axis',(1.,0.,0.));
#18729=DIRECTION('',(1.,0.,0.));
#18730=DIRECTION('',(0.,0.,1.));
#18731=DIRECTION('',(-1.,0.,0.));
#18732=DIRECTION('center_axis',(0.,0.,1.));
#18733=DIRECTION('ref_axis',(-1.,-3.70074341541716E-15,0.));
#18734=DIRECTION('center_axis',(0.,0.,1.));
#18735=DIRECTION('ref_axis',(-1.,-3.70074341541716E-15,0.));
#18736=DIRECTION('center_axis',(0.,0.,-1.));
#18737=DIRECTION('ref_axis',(-1.,-3.70074341541716E-15,0.));
#18738=DIRECTION('center_axis',(-1.,0.,0.));
#18739=DIRECTION('ref_axis',(0.,-1.,0.));
#18740=DIRECTION('',(0.,-1.,0.));
#18741=DIRECTION('',(0.,0.,1.));
#18742=DIRECTION('',(0.,1.,0.));
#18743=DIRECTION('',(0.,0.,1.));
#18744=DIRECTION('center_axis',(0.,0.,1.));
#18745=DIRECTION('ref_axis',(0.,1.,0.));
#18746=DIRECTION('center_axis',(0.,0.,1.));
#18747=DIRECTION('ref_axis',(0.,1.,0.));
#18748=DIRECTION('',(0.,0.,1.));
#18749=DIRECTION('center_axis',(0.,0.,-1.));
#18750=DIRECTION('ref_axis',(0.,1.,0.));
#18751=DIRECTION('center_axis',(0.,1.,0.));
#18752=DIRECTION('ref_axis',(-1.,0.,0.));
#18753=DIRECTION('',(-1.,0.,0.));
#18754=DIRECTION('',(0.,0.,1.));
#18755=DIRECTION('',(1.,0.,0.));
#18756=DIRECTION('center_axis',(0.,0.,1.));
#18757=DIRECTION('ref_axis',(1.,-7.40148683083432E-15,0.));
#18758=DIRECTION('center_axis',(0.,0.,1.));
#18759=DIRECTION('ref_axis',(1.,-7.40148683083432E-15,0.));
#18760=DIRECTION('',(0.,0.,1.));
#18761=DIRECTION('center_axis',(0.,0.,-1.));
#18762=DIRECTION('ref_axis',(1.,-7.40148683083432E-15,0.));
#18763=DIRECTION('center_axis',(1.,0.,0.));
#18764=DIRECTION('ref_axis',(0.,1.,0.));
#18765=DIRECTION('',(0.,1.,0.));
#18766=DIRECTION('',(0.,0.,1.));
#18767=DIRECTION('',(0.,-1.,0.));
#18768=DIRECTION('center_axis',(0.,0.,1.));
#18769=DIRECTION('ref_axis',(0.,-1.,0.));
#18770=DIRECTION('center_axis',(0.,0.,1.));
#18771=DIRECTION('ref_axis',(0.,-1.,0.));
#18772=DIRECTION('',(0.,0.,1.));
#18773=DIRECTION('center_axis',(0.,0.,-1.));
#18774=DIRECTION('ref_axis',(0.,-1.,0.));
#18775=DIRECTION('center_axis',(0.,-1.,0.));
#18776=DIRECTION('ref_axis',(1.,0.,0.));
#18777=DIRECTION('',(1.,0.,0.));
#18778=DIRECTION('',(0.,0.,1.));
#18779=DIRECTION('',(-1.,0.,0.));
#18780=DIRECTION('center_axis',(0.,0.,1.));
#18781=DIRECTION('ref_axis',(-1.,-3.70074341541716E-15,0.));
#18782=DIRECTION('center_axis',(0.,0.,1.));
#18783=DIRECTION('ref_axis',(-1.,-3.70074341541716E-15,0.));
#18784=DIRECTION('center_axis',(0.,0.,-1.));
#18785=DIRECTION('ref_axis',(-1.,-3.70074341541716E-15,0.));
#18786=DIRECTION('center_axis',(-1.,0.,0.));
#18787=DIRECTION('ref_axis',(0.,-1.,0.));
#18788=DIRECTION('',(0.,-1.,0.));
#18789=DIRECTION('',(0.,0.,1.));
#18790=DIRECTION('',(0.,1.,0.));
#18791=DIRECTION('',(0.,0.,1.));
#18792=DIRECTION('center_axis',(0.,0.,1.));
#18793=DIRECTION('ref_axis',(-1.48029736616688E-14,1.,0.));
#18794=DIRECTION('center_axis',(0.,0.,1.));
#18795=DIRECTION('ref_axis',(-1.48029736616688E-14,1.,0.));
#18796=DIRECTION('',(0.,0.,1.));
#18797=DIRECTION('center_axis',(0.,0.,-1.));
#18798=DIRECTION('ref_axis',(-1.48029736616688E-14,1.,0.));
#18799=DIRECTION('center_axis',(0.,1.,0.));
#18800=DIRECTION('ref_axis',(-1.,0.,0.));
#18801=DIRECTION('',(-1.,0.,0.));
#18802=DIRECTION('',(0.,0.,1.));
#18803=DIRECTION('',(1.,0.,0.));
#18804=DIRECTION('center_axis',(0.,0.,1.));
#18805=DIRECTION('ref_axis',(1.,-1.48029736616686E-14,0.));
#18806=DIRECTION('center_axis',(0.,0.,1.));
#18807=DIRECTION('ref_axis',(1.,-1.48029736616686E-14,0.));
#18808=DIRECTION('',(0.,0.,1.));
#18809=DIRECTION('center_axis',(0.,0.,-1.));
#18810=DIRECTION('ref_axis',(1.,-1.48029736616686E-14,0.));
#18811=DIRECTION('center_axis',(1.,0.,0.));
#18812=DIRECTION('ref_axis',(0.,1.,0.));
#18813=DIRECTION('',(0.,1.,0.));
#18814=DIRECTION('',(0.,0.,1.));
#18815=DIRECTION('',(0.,-1.,0.));
#18816=DIRECTION('center_axis',(0.,0.,1.));
#18817=DIRECTION('ref_axis',(1.48029736616688E-14,-1.,0.));
#18818=DIRECTION('center_axis',(0.,0.,1.));
#18819=DIRECTION('ref_axis',(1.48029736616688E-14,-1.,0.));
#18820=DIRECTION('',(0.,0.,1.));
#18821=DIRECTION('center_axis',(0.,0.,-1.));
#18822=DIRECTION('ref_axis',(1.48029736616688E-14,-1.,0.));
#18823=DIRECTION('center_axis',(0.,-1.,0.));
#18824=DIRECTION('ref_axis',(1.,0.,0.));
#18825=DIRECTION('',(1.,0.,0.));
#18826=DIRECTION('',(0.,0.,1.));
#18827=DIRECTION('',(-1.,0.,0.));
#18828=DIRECTION('center_axis',(0.,0.,1.));
#18829=DIRECTION('ref_axis',(-1.,3.70074341541716E-15,0.));
#18830=DIRECTION('center_axis',(0.,0.,1.));
#18831=DIRECTION('ref_axis',(-1.,3.70074341541716E-15,0.));
#18832=DIRECTION('center_axis',(0.,0.,-1.));
#18833=DIRECTION('ref_axis',(-1.,3.70074341541716E-15,0.));
#18834=DIRECTION('center_axis',(-1.,0.,0.));
#18835=DIRECTION('ref_axis',(0.,-1.,0.));
#18836=DIRECTION('',(0.,-1.,0.));
#18837=DIRECTION('',(0.,0.,1.));
#18838=DIRECTION('',(0.,1.,0.));
#18839=DIRECTION('',(0.,0.,1.));
#18840=DIRECTION('center_axis',(0.,0.,1.));
#18841=DIRECTION('ref_axis',(0.,1.,0.));
#18842=DIRECTION('center_axis',(0.,0.,1.));
#18843=DIRECTION('ref_axis',(0.,1.,0.));
#18844=DIRECTION('',(0.,0.,1.));
#18845=DIRECTION('center_axis',(0.,0.,-1.));
#18846=DIRECTION('ref_axis',(0.,1.,0.));
#18847=DIRECTION('center_axis',(0.,1.,0.));
#18848=DIRECTION('ref_axis',(-1.,0.,0.));
#18849=DIRECTION('',(-1.,0.,0.));
#18850=DIRECTION('',(0.,0.,1.));
#18851=DIRECTION('',(1.,0.,0.));
#18852=DIRECTION('center_axis',(0.,0.,1.));
#18853=DIRECTION('ref_axis',(1.,-2.96059473233381E-14,0.));
#18854=DIRECTION('center_axis',(0.,0.,1.));
#18855=DIRECTION('ref_axis',(1.,-2.96059473233381E-14,0.));
#18856=DIRECTION('',(0.,0.,1.));
#18857=DIRECTION('center_axis',(0.,0.,-1.));
#18858=DIRECTION('ref_axis',(1.,-2.96059473233381E-14,0.));
#18859=DIRECTION('center_axis',(1.,0.,0.));
#18860=DIRECTION('ref_axis',(0.,1.,0.));
#18861=DIRECTION('',(0.,1.,0.));
#18862=DIRECTION('',(0.,0.,1.));
#18863=DIRECTION('',(0.,-1.,0.));
#18864=DIRECTION('center_axis',(0.,0.,1.));
#18865=DIRECTION('ref_axis',(0.,-1.,0.));
#18866=DIRECTION('center_axis',(0.,0.,1.));
#18867=DIRECTION('ref_axis',(0.,-1.,0.));
#18868=DIRECTION('',(0.,0.,1.));
#18869=DIRECTION('center_axis',(0.,0.,-1.));
#18870=DIRECTION('ref_axis',(0.,-1.,0.));
#18871=DIRECTION('center_axis',(0.,-1.,0.));
#18872=DIRECTION('ref_axis',(1.,0.,0.));
#18873=DIRECTION('',(1.,0.,0.));
#18874=DIRECTION('',(0.,0.,1.));
#18875=DIRECTION('',(-1.,0.,0.));
#18876=DIRECTION('center_axis',(0.,0.,1.));
#18877=DIRECTION('ref_axis',(-1.,2.22044604925036E-14,0.));
#18878=DIRECTION('center_axis',(0.,0.,1.));
#18879=DIRECTION('ref_axis',(-1.,2.22044604925036E-14,0.));
#18880=DIRECTION('center_axis',(0.,0.,-1.));
#18881=DIRECTION('ref_axis',(-1.,2.22044604925036E-14,0.));
#18882=DIRECTION('center_axis',(-1.,0.,0.));
#18883=DIRECTION('ref_axis',(0.,-1.,0.));
#18884=DIRECTION('',(0.,-1.,0.));
#18885=DIRECTION('',(0.,0.,1.));
#18886=DIRECTION('',(0.,1.,0.));
#18887=DIRECTION('',(0.,0.,1.));
#18888=DIRECTION('center_axis',(0.,0.,1.));
#18889=DIRECTION('ref_axis',(0.,1.,0.));
#18890=DIRECTION('center_axis',(0.,0.,1.));
#18891=DIRECTION('ref_axis',(0.,1.,0.));
#18892=DIRECTION('',(0.,0.,1.));
#18893=DIRECTION('center_axis',(0.,0.,-1.));
#18894=DIRECTION('ref_axis',(0.,1.,0.));
#18895=DIRECTION('center_axis',(0.,1.,0.));
#18896=DIRECTION('ref_axis',(-1.,0.,0.));
#18897=DIRECTION('',(-1.,0.,0.));
#18898=DIRECTION('',(0.,0.,1.));
#18899=DIRECTION('',(1.,0.,0.));
#18900=DIRECTION('center_axis',(0.,0.,1.));
#18901=DIRECTION('ref_axis',(1.,-7.40148683083432E-15,0.));
#18902=DIRECTION('center_axis',(0.,0.,1.));
#18903=DIRECTION('ref_axis',(1.,-7.40148683083432E-15,0.));
#18904=DIRECTION('',(0.,0.,1.));
#18905=DIRECTION('center_axis',(0.,0.,-1.));
#18906=DIRECTION('ref_axis',(1.,-7.40148683083432E-15,0.));
#18907=DIRECTION('center_axis',(1.,0.,0.));
#18908=DIRECTION('ref_axis',(0.,1.,0.));
#18909=DIRECTION('',(0.,1.,0.));
#18910=DIRECTION('',(0.,0.,1.));
#18911=DIRECTION('',(0.,-1.,0.));
#18912=DIRECTION('center_axis',(0.,0.,1.));
#18913=DIRECTION('ref_axis',(0.,-1.,0.));
#18914=DIRECTION('center_axis',(0.,0.,1.));
#18915=DIRECTION('ref_axis',(0.,-1.,0.));
#18916=DIRECTION('',(0.,0.,1.));
#18917=DIRECTION('center_axis',(0.,0.,-1.));
#18918=DIRECTION('ref_axis',(0.,-1.,0.));
#18919=DIRECTION('center_axis',(0.,-1.,0.));
#18920=DIRECTION('ref_axis',(1.,0.,0.));
#18921=DIRECTION('',(1.,0.,0.));
#18922=DIRECTION('',(0.,0.,1.));
#18923=DIRECTION('',(-1.,0.,0.));
#18924=DIRECTION('center_axis',(0.,0.,1.));
#18925=DIRECTION('ref_axis',(-1.,-3.70074341541716E-15,0.));
#18926=DIRECTION('center_axis',(0.,0.,1.));
#18927=DIRECTION('ref_axis',(-1.,-3.70074341541716E-15,0.));
#18928=DIRECTION('center_axis',(0.,0.,-1.));
#18929=DIRECTION('ref_axis',(-1.,-3.70074341541716E-15,0.));
#18930=DIRECTION('center_axis',(-1.,0.,0.));
#18931=DIRECTION('ref_axis',(0.,-1.,0.));
#18932=DIRECTION('',(0.,-1.,0.));
#18933=DIRECTION('',(0.,0.,1.));
#18934=DIRECTION('',(0.,1.,0.));
#18935=DIRECTION('',(0.,0.,1.));
#18936=DIRECTION('center_axis',(0.,0.,1.));
#18937=DIRECTION('ref_axis',(0.,1.,0.));
#18938=DIRECTION('center_axis',(0.,0.,1.));
#18939=DIRECTION('ref_axis',(0.,1.,0.));
#18940=DIRECTION('',(0.,0.,1.));
#18941=DIRECTION('center_axis',(0.,0.,-1.));
#18942=DIRECTION('ref_axis',(0.,1.,0.));
#18943=DIRECTION('center_axis',(0.,1.,0.));
#18944=DIRECTION('ref_axis',(-1.,0.,0.));
#18945=DIRECTION('',(-1.,0.,0.));
#18946=DIRECTION('',(0.,0.,1.));
#18947=DIRECTION('',(1.,0.,0.));
#18948=DIRECTION('center_axis',(0.,0.,1.));
#18949=DIRECTION('ref_axis',(1.,0.,0.));
#18950=DIRECTION('center_axis',(0.,0.,1.));
#18951=DIRECTION('ref_axis',(1.,0.,0.));
#18952=DIRECTION('',(0.,0.,1.));
#18953=DIRECTION('center_axis',(0.,0.,-1.));
#18954=DIRECTION('ref_axis',(1.,0.,0.));
#18955=DIRECTION('center_axis',(1.,0.,0.));
#18956=DIRECTION('ref_axis',(0.,1.,0.));
#18957=DIRECTION('',(0.,1.,0.));
#18958=DIRECTION('',(0.,0.,1.));
#18959=DIRECTION('',(0.,-1.,0.));
#18960=DIRECTION('center_axis',(0.,0.,1.));
#18961=DIRECTION('ref_axis',(2.96059473233373E-14,-1.,0.));
#18962=DIRECTION('center_axis',(0.,0.,1.));
#18963=DIRECTION('ref_axis',(2.96059473233373E-14,-1.,0.));
#18964=DIRECTION('',(0.,0.,1.));
#18965=DIRECTION('center_axis',(0.,0.,-1.));
#18966=DIRECTION('ref_axis',(2.96059473233373E-14,-1.,0.));
#18967=DIRECTION('center_axis',(0.,-1.,0.));
#18968=DIRECTION('ref_axis',(1.,0.,0.));
#18969=DIRECTION('',(1.,0.,0.));
#18970=DIRECTION('',(0.,0.,1.));
#18971=DIRECTION('',(-1.,0.,0.));
#18972=DIRECTION('center_axis',(0.,0.,1.));
#18973=DIRECTION('ref_axis',(-1.,2.22044604925036E-14,0.));
#18974=DIRECTION('center_axis',(0.,0.,1.));
#18975=DIRECTION('ref_axis',(-1.,2.22044604925036E-14,0.));
#18976=DIRECTION('center_axis',(0.,0.,-1.));
#18977=DIRECTION('ref_axis',(-1.,2.22044604925036E-14,0.));
#18978=DIRECTION('center_axis',(-1.,0.,0.));
#18979=DIRECTION('ref_axis',(0.,-1.,0.));
#18980=DIRECTION('',(0.,-1.,0.));
#18981=DIRECTION('',(0.,0.,1.));
#18982=DIRECTION('',(0.,1.,0.));
#18983=DIRECTION('',(0.,0.,1.));
#18984=DIRECTION('center_axis',(0.,0.,1.));
#18985=DIRECTION('ref_axis',(-2.96059473233373E-14,1.,0.));
#18986=DIRECTION('center_axis',(0.,0.,1.));
#18987=DIRECTION('ref_axis',(-2.96059473233373E-14,1.,0.));
#18988=DIRECTION('',(0.,0.,1.));
#18989=DIRECTION('center_axis',(0.,0.,-1.));
#18990=DIRECTION('ref_axis',(-2.96059473233373E-14,1.,0.));
#18991=DIRECTION('center_axis',(0.,1.,0.));
#18992=DIRECTION('ref_axis',(-1.,0.,0.));
#18993=DIRECTION('',(-1.,0.,0.));
#18994=DIRECTION('',(0.,0.,1.));
#18995=DIRECTION('',(1.,0.,0.));
#18996=DIRECTION('center_axis',(0.,0.,1.));
#18997=DIRECTION('ref_axis',(1.,0.,0.));
#18998=DIRECTION('center_axis',(0.,0.,1.));
#18999=DIRECTION('ref_axis',(1.,0.,0.));
#19000=DIRECTION('',(0.,0.,1.));
#19001=DIRECTION('center_axis',(0.,0.,-1.));
#19002=DIRECTION('ref_axis',(1.,0.,0.));
#19003=DIRECTION('center_axis',(1.,0.,0.));
#19004=DIRECTION('ref_axis',(0.,1.,0.));
#19005=DIRECTION('',(0.,1.,0.));
#19006=DIRECTION('',(0.,0.,1.));
#19007=DIRECTION('',(0.,-1.,0.));
#19008=DIRECTION('center_axis',(0.,0.,1.));
#19009=DIRECTION('ref_axis',(2.96059473233373E-14,-1.,0.));
#19010=DIRECTION('center_axis',(0.,0.,1.));
#19011=DIRECTION('ref_axis',(2.96059473233373E-14,-1.,0.));
#19012=DIRECTION('',(0.,0.,1.));
#19013=DIRECTION('center_axis',(0.,0.,-1.));
#19014=DIRECTION('ref_axis',(2.96059473233373E-14,-1.,0.));
#19015=DIRECTION('center_axis',(0.,-1.,0.));
#19016=DIRECTION('ref_axis',(1.,0.,0.));
#19017=DIRECTION('',(1.,0.,0.));
#19018=DIRECTION('',(0.,0.,1.));
#19019=DIRECTION('',(-1.,0.,0.));
#19020=DIRECTION('center_axis',(0.,0.,1.));
#19021=DIRECTION('ref_axis',(-1.,-7.40148683083432E-15,0.));
#19022=DIRECTION('center_axis',(0.,0.,1.));
#19023=DIRECTION('ref_axis',(-1.,-7.40148683083432E-15,0.));
#19024=DIRECTION('center_axis',(0.,0.,-1.));
#19025=DIRECTION('ref_axis',(-1.,-7.40148683083432E-15,0.));
#19026=DIRECTION('center_axis',(-1.,0.,0.));
#19027=DIRECTION('ref_axis',(0.,-1.,0.));
#19028=DIRECTION('',(0.,-1.,0.));
#19029=DIRECTION('',(0.,0.,1.));
#19030=DIRECTION('',(0.,1.,0.));
#19031=DIRECTION('',(0.,0.,1.));
#19032=DIRECTION('center_axis',(0.,0.,1.));
#19033=DIRECTION('ref_axis',(0.,1.,0.));
#19034=DIRECTION('center_axis',(0.,0.,1.));
#19035=DIRECTION('ref_axis',(0.,1.,0.));
#19036=DIRECTION('',(0.,0.,1.));
#19037=DIRECTION('center_axis',(0.,0.,-1.));
#19038=DIRECTION('ref_axis',(0.,1.,0.));
#19039=DIRECTION('center_axis',(0.,1.,0.));
#19040=DIRECTION('ref_axis',(-1.,0.,0.));
#19041=DIRECTION('',(-1.,0.,0.));
#19042=DIRECTION('',(0.,0.,1.));
#19043=DIRECTION('',(1.,0.,0.));
#19044=DIRECTION('center_axis',(0.,0.,1.));
#19045=DIRECTION('ref_axis',(1.,3.70074341541705E-14,0.));
#19046=DIRECTION('center_axis',(0.,0.,1.));
#19047=DIRECTION('ref_axis',(1.,3.70074341541705E-14,0.));
#19048=DIRECTION('',(0.,0.,1.));
#19049=DIRECTION('center_axis',(0.,0.,-1.));
#19050=DIRECTION('ref_axis',(1.,3.70074341541705E-14,0.));
#19051=DIRECTION('center_axis',(1.,0.,0.));
#19052=DIRECTION('ref_axis',(0.,1.,0.));
#19053=DIRECTION('',(0.,1.,0.));
#19054=DIRECTION('',(0.,0.,1.));
#19055=DIRECTION('',(0.,-1.,0.));
#19056=DIRECTION('center_axis',(0.,0.,1.));
#19057=DIRECTION('ref_axis',(0.,-1.,0.));
#19058=DIRECTION('center_axis',(0.,0.,1.));
#19059=DIRECTION('ref_axis',(0.,-1.,0.));
#19060=DIRECTION('',(0.,0.,1.));
#19061=DIRECTION('center_axis',(0.,0.,-1.));
#19062=DIRECTION('ref_axis',(0.,-1.,0.));
#19063=DIRECTION('center_axis',(0.,-1.,0.));
#19064=DIRECTION('ref_axis',(1.,0.,0.));
#19065=DIRECTION('',(1.,0.,0.));
#19066=DIRECTION('',(0.,0.,1.));
#19067=DIRECTION('',(-1.,0.,0.));
#19068=DIRECTION('center_axis',(0.,0.,1.));
#19069=DIRECTION('ref_axis',(-1.,-4.07081775695875E-14,0.));
#19070=DIRECTION('center_axis',(0.,0.,1.));
#19071=DIRECTION('ref_axis',(-1.,-4.07081775695875E-14,0.));
#19072=DIRECTION('center_axis',(0.,0.,-1.));
#19073=DIRECTION('ref_axis',(-1.,-4.07081775695875E-14,0.));
#19074=DIRECTION('center_axis',(-1.,0.,0.));
#19075=DIRECTION('ref_axis',(0.,-1.,0.));
#19076=DIRECTION('',(0.,-1.,0.));
#19077=DIRECTION('',(0.,0.,1.));
#19078=DIRECTION('',(0.,-1.,0.));
#19079=DIRECTION('',(0.,0.,1.));
#19080=DIRECTION('center_axis',(0.,0.,1.));
#19081=DIRECTION('ref_axis',(0.,1.,0.));
#19082=DIRECTION('center_axis',(0.,0.,1.));
#19083=DIRECTION('ref_axis',(0.,1.,0.));
#19084=DIRECTION('center_axis',(0.,0.,1.));
#19085=DIRECTION('ref_axis',(0.,1.,0.));
#19086=DIRECTION('',(0.,0.,1.));
#19087=DIRECTION('center_axis',(0.,1.,0.));
#19088=DIRECTION('ref_axis',(-1.,0.,0.));
#19089=DIRECTION('',(-1.,0.,0.));
#19090=DIRECTION('',(-1.,0.,0.));
#19091=DIRECTION('',(0.,0.,1.));
#19092=DIRECTION('center_axis',(0.,0.,1.));
#19093=DIRECTION('ref_axis',(1.,8.88178419700113E-15,0.));
#19094=DIRECTION('center_axis',(0.,0.,1.));
#19095=DIRECTION('ref_axis',(1.,8.88178419700113E-15,0.));
#19096=DIRECTION('center_axis',(0.,0.,1.));
#19097=DIRECTION('ref_axis',(1.,8.88178419700113E-15,0.));
#19098=DIRECTION('',(0.,0.,1.));
#19099=DIRECTION('center_axis',(1.,0.,0.));
#19100=DIRECTION('ref_axis',(0.,1.,0.));
#19101=DIRECTION('',(0.,1.,0.));
#19102=DIRECTION('',(0.,1.,0.));
#19103=DIRECTION('',(0.,0.,1.));
#19104=DIRECTION('center_axis',(0.,0.,1.));
#19105=DIRECTION('ref_axis',(0.,-1.,0.));
#19106=DIRECTION('center_axis',(0.,0.,1.));
#19107=DIRECTION('ref_axis',(0.,-1.,0.));
#19108=DIRECTION('center_axis',(0.,0.,1.));
#19109=DIRECTION('ref_axis',(0.,-1.,0.));
#19110=DIRECTION('',(0.,0.,1.));
#19111=DIRECTION('center_axis',(0.,-1.,0.));
#19112=DIRECTION('ref_axis',(1.,0.,0.));
#19113=DIRECTION('',(1.,0.,0.));
#19114=DIRECTION('',(1.,0.,0.));
#19115=DIRECTION('',(0.,0.,1.));
#19116=DIRECTION('center_axis',(0.,0.,1.));
#19117=DIRECTION('ref_axis',(-1.,-2.22044604925031E-15,0.));
#19118=DIRECTION('center_axis',(0.,0.,1.));
#19119=DIRECTION('ref_axis',(-1.,-2.22044604925031E-15,0.));
#19120=DIRECTION('center_axis',(0.,0.,1.));
#19121=DIRECTION('ref_axis',(-1.,-2.22044604925031E-15,0.));
#19122=DIRECTION('center_axis',(0.,0.,1.));
#19123=DIRECTION('ref_axis',(1.,0.,0.));
#19124=DIRECTION('center_axis',(0.,0.,1.));
#19125=DIRECTION('ref_axis',(1.,0.,0.));
#22246=CARTESIAN_POINT('',(0.,0.,0.));
#22247=CARTESIAN_POINT('Origin',(169.2,22.1,31.45));
#22248=CARTESIAN_POINT('',(169.2,22.1,31.45));
#22249=CARTESIAN_POINT('',(169.2,19.9,31.45));
#22250=CARTESIAN_POINT('',(169.2,21.55,31.45));
#22251=CARTESIAN_POINT('',(169.2,22.1,32.55));
#22252=CARTESIAN_POINT('',(169.2,22.1,31.45));
#22253=CARTESIAN_POINT('',(169.2,19.9,32.55));
#22254=CARTESIAN_POINT('',(169.2,21.55,32.55));
#22255=CARTESIAN_POINT('',(169.2,19.9,31.45));
#22256=CARTESIAN_POINT('Origin',(169.6,22.1,31.45));
#22257=CARTESIAN_POINT('',(169.6,22.5,31.45));
#22258=CARTESIAN_POINT('Origin',(169.6,22.1,31.45));
#22259=CARTESIAN_POINT('',(169.6,22.5,32.55));
#22260=CARTESIAN_POINT('',(169.6,22.5,31.45));
#22261=CARTESIAN_POINT('Origin',(169.6,22.1,32.55));
#22262=CARTESIAN_POINT('Origin',(170.,22.5,31.45));
#22263=CARTESIAN_POINT('',(170.,22.5,31.45));
#22264=CARTESIAN_POINT('',(137.5,22.5,31.45));
#22265=CARTESIAN_POINT('',(170.,22.5,32.55));
#22266=CARTESIAN_POINT('',(170.,22.5,31.45));
#22267=CARTESIAN_POINT('',(137.5,22.5,32.55));
#22268=CARTESIAN_POINT('Origin',(170.,22.1000000000001,31.45));
#22269=CARTESIAN_POINT('',(170.4,22.1,31.45));
#22270=CARTESIAN_POINT('Origin',(170.,22.1000000000001,31.45));
#22271=CARTESIAN_POINT('',(170.4,22.1,32.55));
#22272=CARTESIAN_POINT('',(170.4,22.1,31.45));
#22273=CARTESIAN_POINT('Origin',(170.,22.1000000000001,32.55));
#22274=CARTESIAN_POINT('Origin',(170.4,19.9,31.45));
#22275=CARTESIAN_POINT('',(170.4,19.9,31.45));
#22276=CARTESIAN_POINT('',(170.4,20.45,31.45));
#22277=CARTESIAN_POINT('',(170.4,19.9,32.55));
#22278=CARTESIAN_POINT('',(170.4,19.9,31.45));
#22279=CARTESIAN_POINT('',(170.4,20.45,32.55));
#22280=CARTESIAN_POINT('Origin',(170.,19.8999999999999,31.45));
#22281=CARTESIAN_POINT('',(170.,19.5,31.45));
#22282=CARTESIAN_POINT('Origin',(170.,19.8999999999999,31.45));
#22283=CARTESIAN_POINT('',(170.,19.5,32.55));
#22284=CARTESIAN_POINT('',(170.,19.5,31.45));
#22285=CARTESIAN_POINT('Origin',(170.,19.8999999999999,32.55));
#22286=CARTESIAN_POINT('Origin',(169.6,19.5,31.45));
#22287=CARTESIAN_POINT('',(169.6,19.5,31.45));
#22288=CARTESIAN_POINT('',(137.3,19.5,31.45));
#22289=CARTESIAN_POINT('',(169.6,19.5,32.55));
#22290=CARTESIAN_POINT('',(169.6,19.5,31.45));
#22291=CARTESIAN_POINT('',(137.3,19.5,32.55));
#22292=CARTESIAN_POINT('Origin',(169.6,19.9,31.45));
#22293=CARTESIAN_POINT('Origin',(169.6,19.9,31.45));
#22294=CARTESIAN_POINT('Origin',(169.6,19.9,32.55));
#22295=CARTESIAN_POINT('Origin',(39.6,22.1,31.45));
#22296=CARTESIAN_POINT('',(39.6,22.1,31.45));
#22297=CARTESIAN_POINT('',(39.6,19.9,31.45));
#22298=CARTESIAN_POINT('',(39.6,21.55,31.45));
#22299=CARTESIAN_POINT('',(39.6,22.1,32.55));
#22300=CARTESIAN_POINT('',(39.6,22.1,31.45));
#22301=CARTESIAN_POINT('',(39.6,19.9,32.55));
#22302=CARTESIAN_POINT('',(39.6,21.55,32.55));
#22303=CARTESIAN_POINT('',(39.6,19.9,31.45));
#22304=CARTESIAN_POINT('Origin',(40.,22.1,31.45));
#22305=CARTESIAN_POINT('',(40.,22.5,31.45));
#22306=CARTESIAN_POINT('Origin',(40.,22.1,31.45));
#22307=CARTESIAN_POINT('',(40.,22.5,32.55));
#22308=CARTESIAN_POINT('',(40.,22.5,31.45));
#22309=CARTESIAN_POINT('Origin',(40.,22.1,32.55));
#22310=CARTESIAN_POINT('Origin',(40.4,22.5,31.45));
#22311=CARTESIAN_POINT('',(40.4,22.5,31.45));
#22312=CARTESIAN_POINT('',(72.7,22.5,31.45));
#22313=CARTESIAN_POINT('',(40.4,22.5,32.55));
#22314=CARTESIAN_POINT('',(40.4,22.5,31.45));
#22315=CARTESIAN_POINT('',(72.7,22.5,32.55));
#22316=CARTESIAN_POINT('Origin',(40.4,22.1,31.45));
#22317=CARTESIAN_POINT('',(40.8,22.1,31.45));
#22318=CARTESIAN_POINT('Origin',(40.4,22.1,31.45));
#22319=CARTESIAN_POINT('',(40.8,22.1,32.55));
#22320=CARTESIAN_POINT('',(40.8,22.1,31.45));
#22321=CARTESIAN_POINT('Origin',(40.4,22.1,32.55));
#22322=CARTESIAN_POINT('Origin',(40.8,19.9,31.45));
#22323=CARTESIAN_POINT('',(40.8,19.9,31.45));
#22324=CARTESIAN_POINT('',(40.8,20.45,31.45));
#22325=CARTESIAN_POINT('',(40.8,19.9,32.55));
#22326=CARTESIAN_POINT('',(40.8,19.9,31.45));
#22327=CARTESIAN_POINT('',(40.8,20.45,32.55));
#22328=CARTESIAN_POINT('Origin',(40.4,19.9,31.45));
#22329=CARTESIAN_POINT('',(40.4,19.5,31.45));
#22330=CARTESIAN_POINT('Origin',(40.4,19.9,31.45));
#22331=CARTESIAN_POINT('',(40.4,19.5,32.55));
#22332=CARTESIAN_POINT('',(40.4,19.5,31.45));
#22333=CARTESIAN_POINT('Origin',(40.4,19.9,32.55));
#22334=CARTESIAN_POINT('Origin',(40.,19.5,31.45));
#22335=CARTESIAN_POINT('',(40.,19.5,31.45));
#22336=CARTESIAN_POINT('',(72.5,19.5,31.45));
#22337=CARTESIAN_POINT('',(40.,19.5,32.55));
#22338=CARTESIAN_POINT('',(40.,19.5,31.45));
#22339=CARTESIAN_POINT('',(72.5,19.5,32.55));
#22340=CARTESIAN_POINT('Origin',(40.,19.9,31.45));
#22341=CARTESIAN_POINT('Origin',(40.,19.9,31.45));
#22342=CARTESIAN_POINT('Origin',(40.,19.9,32.55));
#22343=CARTESIAN_POINT('Origin',(151.8,24.7,31.45));
#22344=CARTESIAN_POINT('',(151.8,24.7,31.45));
#22345=CARTESIAN_POINT('',(151.8,17.3,31.45));
#22346=CARTESIAN_POINT('',(151.8,22.85,31.45));
#22347=CARTESIAN_POINT('',(151.8,24.7,32.55));
#22348=CARTESIAN_POINT('',(151.8,24.7,31.45));
#22349=CARTESIAN_POINT('',(151.8,17.3,32.55));
#22350=CARTESIAN_POINT('',(151.8,22.85,32.55));
#22351=CARTESIAN_POINT('',(151.8,17.3,31.45));
#22352=CARTESIAN_POINT('Origin',(152.4,24.7,31.45));
#22353=CARTESIAN_POINT('',(152.4,25.3,31.45));
#22354=CARTESIAN_POINT('Origin',(152.4,24.7,31.45));
#22355=CARTESIAN_POINT('',(152.4,25.3,32.55));
#22356=CARTESIAN_POINT('',(152.4,25.3,31.45));
#22357=CARTESIAN_POINT('Origin',(152.4,24.7,32.55));
#22358=CARTESIAN_POINT('Origin',(157.6,25.3,31.45));
#22359=CARTESIAN_POINT('',(157.6,25.3,31.45));
#22360=CARTESIAN_POINT('',(131.3,25.3,31.45));
#22361=CARTESIAN_POINT('',(157.6,25.3,32.55));
#22362=CARTESIAN_POINT('',(157.6,25.3,31.45));
#22363=CARTESIAN_POINT('',(131.3,25.3,32.55));
#22364=CARTESIAN_POINT('Origin',(157.6,24.7,31.45));
#22365=CARTESIAN_POINT('',(158.2,24.7,31.45));
#22366=CARTESIAN_POINT('Origin',(157.6,24.7,31.45));
#22367=CARTESIAN_POINT('',(158.2,24.7,32.55));
#22368=CARTESIAN_POINT('',(158.2,24.7,31.45));
#22369=CARTESIAN_POINT('Origin',(157.6,24.7,32.55));
#22370=CARTESIAN_POINT('Origin',(158.2,17.3,31.45));
#22371=CARTESIAN_POINT('',(158.2,17.3,31.45));
#22372=CARTESIAN_POINT('',(158.2,19.15,31.45));
#22373=CARTESIAN_POINT('',(158.2,17.3,32.55));
#22374=CARTESIAN_POINT('',(158.2,17.3,31.45));
#22375=CARTESIAN_POINT('',(158.2,19.15,32.55));
#22376=CARTESIAN_POINT('Origin',(157.6,17.3,31.45));
#22377=CARTESIAN_POINT('',(157.6,16.7,31.45));
#22378=CARTESIAN_POINT('Origin',(157.6,17.3,31.45));
#22379=CARTESIAN_POINT('',(157.6,16.7,32.55));
#22380=CARTESIAN_POINT('',(157.6,16.7,31.45));
#22381=CARTESIAN_POINT('Origin',(157.6,17.3,32.55));
#22382=CARTESIAN_POINT('Origin',(152.4,16.7,31.45));
#22383=CARTESIAN_POINT('',(152.4,16.7,31.45));
#22384=CARTESIAN_POINT('',(128.7,16.7,31.45));
#22385=CARTESIAN_POINT('',(152.4,16.7,32.55));
#22386=CARTESIAN_POINT('',(152.4,16.7,31.45));
#22387=CARTESIAN_POINT('',(128.7,16.7,32.55));
#22388=CARTESIAN_POINT('Origin',(152.4,17.3,31.45));
#22389=CARTESIAN_POINT('Origin',(152.4,17.3,31.45));
#22390=CARTESIAN_POINT('Origin',(152.4,17.3,32.55));
#22391=CARTESIAN_POINT('Origin',(131.8,24.7,31.45));
#22392=CARTESIAN_POINT('',(131.8,24.7,31.45));
#22393=CARTESIAN_POINT('',(131.8,17.3,31.45));
#22394=CARTESIAN_POINT('',(131.8,22.85,31.45));
#22395=CARTESIAN_POINT('',(131.8,24.7,32.55));
#22396=CARTESIAN_POINT('',(131.8,24.7,31.45));
#22397=CARTESIAN_POINT('',(131.8,17.3,32.55));
#22398=CARTESIAN_POINT('',(131.8,22.85,32.55));
#22399=CARTESIAN_POINT('',(131.8,17.3,31.45));
#22400=CARTESIAN_POINT('Origin',(132.4,24.7,31.45));
#22401=CARTESIAN_POINT('',(132.4,25.3,31.45));
#22402=CARTESIAN_POINT('Origin',(132.4,24.7,31.45));
#22403=CARTESIAN_POINT('',(132.4,25.3,32.55));
#22404=CARTESIAN_POINT('',(132.4,25.3,31.45));
#22405=CARTESIAN_POINT('Origin',(132.4,24.7,32.55));
#22406=CARTESIAN_POINT('Origin',(137.6,25.3,31.45));
#22407=CARTESIAN_POINT('',(137.6,25.3,31.45));
#22408=CARTESIAN_POINT('',(121.3,25.3,31.45));
#22409=CARTESIAN_POINT('',(137.6,25.3,32.55));
#22410=CARTESIAN_POINT('',(137.6,25.3,31.45));
#22411=CARTESIAN_POINT('',(121.3,25.3,32.55));
#22412=CARTESIAN_POINT('Origin',(137.6,24.7,31.45));
#22413=CARTESIAN_POINT('',(138.2,24.7,31.45));
#22414=CARTESIAN_POINT('Origin',(137.6,24.7,31.45));
#22415=CARTESIAN_POINT('',(138.2,24.7,32.55));
#22416=CARTESIAN_POINT('',(138.2,24.7,31.45));
#22417=CARTESIAN_POINT('Origin',(137.6,24.7,32.55));
#22418=CARTESIAN_POINT('Origin',(138.2,17.3,31.45));
#22419=CARTESIAN_POINT('',(138.2,17.3,31.45));
#22420=CARTESIAN_POINT('',(138.2,19.15,31.45));
#22421=CARTESIAN_POINT('',(138.2,17.3,32.55));
#22422=CARTESIAN_POINT('',(138.2,17.3,31.45));
#22423=CARTESIAN_POINT('',(138.2,19.15,32.55));
#22424=CARTESIAN_POINT('Origin',(137.6,17.3,31.45));
#22425=CARTESIAN_POINT('',(137.6,16.7,31.45));
#22426=CARTESIAN_POINT('Origin',(137.6,17.3,31.45));
#22427=CARTESIAN_POINT('',(137.6,16.7,32.55));
#22428=CARTESIAN_POINT('',(137.6,16.7,31.45));
#22429=CARTESIAN_POINT('Origin',(137.6,17.3,32.55));
#22430=CARTESIAN_POINT('Origin',(132.4,16.7,31.45));
#22431=CARTESIAN_POINT('',(132.4,16.7,31.45));
#22432=CARTESIAN_POINT('',(118.7,16.7,31.45));
#22433=CARTESIAN_POINT('',(132.4,16.7,32.55));
#22434=CARTESIAN_POINT('',(132.4,16.7,31.45));
#22435=CARTESIAN_POINT('',(118.7,16.7,32.55));
#22436=CARTESIAN_POINT('Origin',(132.4,17.3,31.45));
#22437=CARTESIAN_POINT('Origin',(132.4,17.3,31.45));
#22438=CARTESIAN_POINT('Origin',(132.4,17.3,32.55));
#22439=CARTESIAN_POINT('Origin',(111.8,24.7,31.45));
#22440=CARTESIAN_POINT('',(111.8,24.7,31.45));
#22441=CARTESIAN_POINT('',(111.8,17.3,31.45));
#22442=CARTESIAN_POINT('',(111.8,22.85,31.45));
#22443=CARTESIAN_POINT('',(111.8,24.7,32.55));
#22444=CARTESIAN_POINT('',(111.8,24.7,31.45));
#22445=CARTESIAN_POINT('',(111.8,17.3,32.55));
#22446=CARTESIAN_POINT('',(111.8,22.85,32.55));
#22447=CARTESIAN_POINT('',(111.8,17.3,31.45));
#22448=CARTESIAN_POINT('Origin',(112.4,24.7,31.45));
#22449=CARTESIAN_POINT('',(112.4,25.3,31.45));
#22450=CARTESIAN_POINT('Origin',(112.4,24.7,31.45));
#22451=CARTESIAN_POINT('',(112.4,25.3,32.55));
#22452=CARTESIAN_POINT('',(112.4,25.3,31.45));
#22453=CARTESIAN_POINT('Origin',(112.4,24.7,32.55));
#22454=CARTESIAN_POINT('Origin',(117.6,25.3,31.45));
#22455=CARTESIAN_POINT('',(117.6,25.3,31.45));
#22456=CARTESIAN_POINT('',(111.3,25.3,31.45));
#22457=CARTESIAN_POINT('',(117.6,25.3,32.55));
#22458=CARTESIAN_POINT('',(117.6,25.3,31.45));
#22459=CARTESIAN_POINT('',(111.3,25.3,32.55));
#22460=CARTESIAN_POINT('Origin',(117.6,24.7,31.45));
#22461=CARTESIAN_POINT('',(118.2,24.7,31.45));
#22462=CARTESIAN_POINT('Origin',(117.6,24.7,31.45));
#22463=CARTESIAN_POINT('',(118.2,24.7,32.55));
#22464=CARTESIAN_POINT('',(118.2,24.7,31.45));
#22465=CARTESIAN_POINT('Origin',(117.6,24.7,32.55));
#22466=CARTESIAN_POINT('Origin',(118.2,17.3,31.45));
#22467=CARTESIAN_POINT('',(118.2,17.3,31.45));
#22468=CARTESIAN_POINT('',(118.2,19.15,31.45));
#22469=CARTESIAN_POINT('',(118.2,17.3,32.55));
#22470=CARTESIAN_POINT('',(118.2,17.3,31.45));
#22471=CARTESIAN_POINT('',(118.2,19.15,32.55));
#22472=CARTESIAN_POINT('Origin',(117.6,17.3,31.45));
#22473=CARTESIAN_POINT('',(117.6,16.7,31.45));
#22474=CARTESIAN_POINT('Origin',(117.6,17.3,31.45));
#22475=CARTESIAN_POINT('',(117.6,16.7,32.55));
#22476=CARTESIAN_POINT('',(117.6,16.7,31.45));
#22477=CARTESIAN_POINT('Origin',(117.6,17.3,32.55));
#22478=CARTESIAN_POINT('Origin',(112.4,16.7,31.45));
#22479=CARTESIAN_POINT('',(112.4,16.7,31.45));
#22480=CARTESIAN_POINT('',(108.7,16.7,31.45));
#22481=CARTESIAN_POINT('',(112.4,16.7,32.55));
#22482=CARTESIAN_POINT('',(112.4,16.7,31.45));
#22483=CARTESIAN_POINT('',(108.7,16.7,32.55));
#22484=CARTESIAN_POINT('Origin',(112.4,17.3,31.45));
#22485=CARTESIAN_POINT('Origin',(112.4,17.3,31.45));
#22486=CARTESIAN_POINT('Origin',(112.4,17.3,32.55));
#22487=CARTESIAN_POINT('Origin',(101.8,24.7,31.45));
#22488=CARTESIAN_POINT('',(101.8,24.7,31.45));
#22489=CARTESIAN_POINT('',(101.8,17.3,31.45));
#22490=CARTESIAN_POINT('',(101.8,22.85,31.45));
#22491=CARTESIAN_POINT('',(101.8,24.7,32.55));
#22492=CARTESIAN_POINT('',(101.8,24.7,31.45));
#22493=CARTESIAN_POINT('',(101.8,17.3,32.55));
#22494=CARTESIAN_POINT('',(101.8,22.85,32.55));
#22495=CARTESIAN_POINT('',(101.8,17.3,31.45));
#22496=CARTESIAN_POINT('Origin',(102.4,24.7,31.45));
#22497=CARTESIAN_POINT('',(102.4,25.3,31.45));
#22498=CARTESIAN_POINT('Origin',(102.4,24.7,31.45));
#22499=CARTESIAN_POINT('',(102.4,25.3,32.55));
#22500=CARTESIAN_POINT('',(102.4,25.3,31.45));
#22501=CARTESIAN_POINT('Origin',(102.4,24.7,32.55));
#22502=CARTESIAN_POINT('Origin',(107.6,25.3,31.45));
#22503=CARTESIAN_POINT('',(107.6,25.3,31.45));
#22504=CARTESIAN_POINT('',(106.3,25.3,31.45));
#22505=CARTESIAN_POINT('',(107.6,25.3,32.55));
#22506=CARTESIAN_POINT('',(107.6,25.3,31.45));
#22507=CARTESIAN_POINT('',(106.3,25.3,32.55));
#22508=CARTESIAN_POINT('Origin',(107.6,24.7,31.45));
#22509=CARTESIAN_POINT('',(108.2,24.7,31.45));
#22510=CARTESIAN_POINT('Origin',(107.6,24.7,31.45));
#22511=CARTESIAN_POINT('',(108.2,24.7,32.55));
#22512=CARTESIAN_POINT('',(108.2,24.7,31.45));
#22513=CARTESIAN_POINT('Origin',(107.6,24.7,32.55));
#22514=CARTESIAN_POINT('Origin',(108.2,17.3,31.45));
#22515=CARTESIAN_POINT('',(108.2,17.3,31.45));
#22516=CARTESIAN_POINT('',(108.2,19.15,31.45));
#22517=CARTESIAN_POINT('',(108.2,17.3,32.55));
#22518=CARTESIAN_POINT('',(108.2,17.3,31.45));
#22519=CARTESIAN_POINT('',(108.2,19.15,32.55));
#22520=CARTESIAN_POINT('Origin',(107.6,17.3,31.45));
#22521=CARTESIAN_POINT('',(107.6,16.7,31.45));
#22522=CARTESIAN_POINT('Origin',(107.6,17.3,31.45));
#22523=CARTESIAN_POINT('',(107.6,16.7,32.55));
#22524=CARTESIAN_POINT('',(107.6,16.7,31.45));
#22525=CARTESIAN_POINT('Origin',(107.6,17.3,32.55));
#22526=CARTESIAN_POINT('Origin',(102.4,16.7,31.45));
#22527=CARTESIAN_POINT('',(102.4,16.7,31.45));
#22528=CARTESIAN_POINT('',(103.7,16.7,31.45));
#22529=CARTESIAN_POINT('',(102.4,16.7,32.55));
#22530=CARTESIAN_POINT('',(102.4,16.7,31.45));
#22531=CARTESIAN_POINT('',(103.7,16.7,32.55));
#22532=CARTESIAN_POINT('Origin',(102.4,17.3,31.45));
#22533=CARTESIAN_POINT('Origin',(102.4,17.3,31.45));
#22534=CARTESIAN_POINT('Origin',(102.4,17.3,32.55));
#22535=CARTESIAN_POINT('Origin',(81.8,24.7,31.45));
#22536=CARTESIAN_POINT('',(81.8,24.7,31.45));
#22537=CARTESIAN_POINT('',(81.8,17.3,31.45));
#22538=CARTESIAN_POINT('',(81.8,22.85,31.45));
#22539=CARTESIAN_POINT('',(81.8,24.7,32.55));
#22540=CARTESIAN_POINT('',(81.8,24.7,31.45));
#22541=CARTESIAN_POINT('',(81.8,17.3,32.55));
#22542=CARTESIAN_POINT('',(81.8,22.85,32.55));
#22543=CARTESIAN_POINT('',(81.8,17.3,31.45));
#22544=CARTESIAN_POINT('Origin',(82.4,24.7,31.45));
#22545=CARTESIAN_POINT('',(82.4,25.3,31.45));
#22546=CARTESIAN_POINT('Origin',(82.4,24.7,31.45));
#22547=CARTESIAN_POINT('',(82.4,25.3,32.55));
#22548=CARTESIAN_POINT('',(82.4,25.3,31.45));
#22549=CARTESIAN_POINT('Origin',(82.4,24.7,32.55));
#22550=CARTESIAN_POINT('Origin',(87.6,25.3,31.45));
#22551=CARTESIAN_POINT('',(87.6,25.3,31.45));
#22552=CARTESIAN_POINT('',(96.3,25.3,31.45));
#22553=CARTESIAN_POINT('',(87.6,25.3,32.55));
#22554=CARTESIAN_POINT('',(87.6,25.3,31.45));
#22555=CARTESIAN_POINT('',(96.3,25.3,32.55));
#22556=CARTESIAN_POINT('Origin',(87.6,24.7,31.45));
#22557=CARTESIAN_POINT('',(88.2,24.7,31.45));
#22558=CARTESIAN_POINT('Origin',(87.6,24.7,31.45));
#22559=CARTESIAN_POINT('',(88.2,24.7,32.55));
#22560=CARTESIAN_POINT('',(88.2,24.7,31.45));
#22561=CARTESIAN_POINT('Origin',(87.6,24.7,32.55));
#22562=CARTESIAN_POINT('Origin',(88.2,17.3,31.45));
#22563=CARTESIAN_POINT('',(88.2,17.3,31.45));
#22564=CARTESIAN_POINT('',(88.2,19.15,31.45));
#22565=CARTESIAN_POINT('',(88.2,17.3,32.55));
#22566=CARTESIAN_POINT('',(88.2,17.3,31.45));
#22567=CARTESIAN_POINT('',(88.2,19.15,32.55));
#22568=CARTESIAN_POINT('Origin',(87.6,17.3,31.45));
#22569=CARTESIAN_POINT('',(87.6,16.7,31.45));
#22570=CARTESIAN_POINT('Origin',(87.6,17.3,31.45));
#22571=CARTESIAN_POINT('',(87.6,16.7,32.55));
#22572=CARTESIAN_POINT('',(87.6,16.7,31.45));
#22573=CARTESIAN_POINT('Origin',(87.6,17.3,32.55));
#22574=CARTESIAN_POINT('Origin',(82.4,16.7,31.45));
#22575=CARTESIAN_POINT('',(82.4,16.7,31.45));
#22576=CARTESIAN_POINT('',(93.7,16.7,31.45));
#22577=CARTESIAN_POINT('',(82.4,16.7,32.55));
#22578=CARTESIAN_POINT('',(82.4,16.7,31.45));
#22579=CARTESIAN_POINT('',(93.7,16.7,32.55));
#22580=CARTESIAN_POINT('Origin',(82.4,17.3,31.45));
#22581=CARTESIAN_POINT('Origin',(82.4,17.3,31.45));
#22582=CARTESIAN_POINT('Origin',(82.4,17.3,32.55));
#22583=CARTESIAN_POINT('Origin',(61.8,24.7,31.45));
#22584=CARTESIAN_POINT('',(61.8,24.7,31.45));
#22585=CARTESIAN_POINT('',(61.8,17.3,31.45));
#22586=CARTESIAN_POINT('',(61.8,22.85,31.45));
#22587=CARTESIAN_POINT('',(61.8,24.7,32.55));
#22588=CARTESIAN_POINT('',(61.8,24.7,31.45));
#22589=CARTESIAN_POINT('',(61.8,17.3,32.55));
#22590=CARTESIAN_POINT('',(61.8,22.85,32.55));
#22591=CARTESIAN_POINT('',(61.8,17.3,31.45));
#22592=CARTESIAN_POINT('Origin',(62.4,24.7,31.45));
#22593=CARTESIAN_POINT('',(62.4,25.3,31.45));
#22594=CARTESIAN_POINT('Origin',(62.4,24.7,31.45));
#22595=CARTESIAN_POINT('',(62.4,25.3,32.55));
#22596=CARTESIAN_POINT('',(62.4,25.3,31.45));
#22597=CARTESIAN_POINT('Origin',(62.4,24.7,32.55));
#22598=CARTESIAN_POINT('Origin',(67.6,25.3,31.45));
#22599=CARTESIAN_POINT('',(67.6,25.3,31.45));
#22600=CARTESIAN_POINT('',(86.3,25.3,31.45));
#22601=CARTESIAN_POINT('',(67.6,25.3,32.55));
#22602=CARTESIAN_POINT('',(67.6,25.3,31.45));
#22603=CARTESIAN_POINT('',(86.3,25.3,32.55));
#22604=CARTESIAN_POINT('Origin',(67.6,24.7,31.45));
#22605=CARTESIAN_POINT('',(68.2,24.7,31.45));
#22606=CARTESIAN_POINT('Origin',(67.6,24.7,31.45));
#22607=CARTESIAN_POINT('',(68.2,24.7,32.55));
#22608=CARTESIAN_POINT('',(68.2,24.7,31.45));
#22609=CARTESIAN_POINT('Origin',(67.6,24.7,32.55));
#22610=CARTESIAN_POINT('Origin',(68.2,17.3,31.45));
#22611=CARTESIAN_POINT('',(68.2,17.3,31.45));
#22612=CARTESIAN_POINT('',(68.2,19.15,31.45));
#22613=CARTESIAN_POINT('',(68.2,17.3,32.55));
#22614=CARTESIAN_POINT('',(68.2,17.3,31.45));
#22615=CARTESIAN_POINT('',(68.2,19.15,32.55));
#22616=CARTESIAN_POINT('Origin',(67.6,17.3,31.45));
#22617=CARTESIAN_POINT('',(67.6,16.7,31.45));
#22618=CARTESIAN_POINT('Origin',(67.6,17.3,31.45));
#22619=CARTESIAN_POINT('',(67.6,16.7,32.55));
#22620=CARTESIAN_POINT('',(67.6,16.7,31.45));
#22621=CARTESIAN_POINT('Origin',(67.6,17.3,32.55));
#22622=CARTESIAN_POINT('Origin',(62.4,16.7,31.45));
#22623=CARTESIAN_POINT('',(62.4,16.7,31.45));
#22624=CARTESIAN_POINT('',(83.7,16.7,31.45));
#22625=CARTESIAN_POINT('',(62.4,16.7,32.55));
#22626=CARTESIAN_POINT('',(62.4,16.7,31.45));
#22627=CARTESIAN_POINT('',(83.7,16.7,32.55));
#22628=CARTESIAN_POINT('Origin',(62.4,17.3,31.45));
#22629=CARTESIAN_POINT('Origin',(62.4,17.3,31.45));
#22630=CARTESIAN_POINT('Origin',(62.4,17.3,32.55));
#22631=CARTESIAN_POINT('Origin',(51.8,24.7,31.45));
#22632=CARTESIAN_POINT('',(51.8,24.7,31.45));
#22633=CARTESIAN_POINT('',(51.8,17.3,31.45));
#22634=CARTESIAN_POINT('',(51.8,22.85,31.45));
#22635=CARTESIAN_POINT('',(51.8,24.7,32.55));
#22636=CARTESIAN_POINT('',(51.8,24.7,31.45));
#22637=CARTESIAN_POINT('',(51.8,17.3,32.55));
#22638=CARTESIAN_POINT('',(51.8,22.85,32.55));
#22639=CARTESIAN_POINT('',(51.8,17.3,31.45));
#22640=CARTESIAN_POINT('Origin',(52.4,24.7,31.45));
#22641=CARTESIAN_POINT('',(52.4,25.3,31.45));
#22642=CARTESIAN_POINT('Origin',(52.4,24.7,31.45));
#22643=CARTESIAN_POINT('',(52.4,25.3,32.55));
#22644=CARTESIAN_POINT('',(52.4,25.3,31.45));
#22645=CARTESIAN_POINT('Origin',(52.4,24.7,32.55));
#22646=CARTESIAN_POINT('Origin',(57.6,25.3,31.45));
#22647=CARTESIAN_POINT('',(57.6,25.3,31.45));
#22648=CARTESIAN_POINT('',(81.3,25.3,31.45));
#22649=CARTESIAN_POINT('',(57.6,25.3,32.55));
#22650=CARTESIAN_POINT('',(57.6,25.3,31.45));
#22651=CARTESIAN_POINT('',(81.3,25.3,32.55));
#22652=CARTESIAN_POINT('Origin',(57.6,24.7,31.45));
#22653=CARTESIAN_POINT('',(58.2,24.7,31.45));
#22654=CARTESIAN_POINT('Origin',(57.6,24.7,31.45));
#22655=CARTESIAN_POINT('',(58.2,24.7,32.55));
#22656=CARTESIAN_POINT('',(58.2,24.7,31.45));
#22657=CARTESIAN_POINT('Origin',(57.6,24.7,32.55));
#22658=CARTESIAN_POINT('Origin',(58.2,17.3,31.45));
#22659=CARTESIAN_POINT('',(58.2,17.3,31.45));
#22660=CARTESIAN_POINT('',(58.2,19.15,31.45));
#22661=CARTESIAN_POINT('',(58.2,17.3,32.55));
#22662=CARTESIAN_POINT('',(58.2,17.3,31.45));
#22663=CARTESIAN_POINT('',(58.2,19.15,32.55));
#22664=CARTESIAN_POINT('Origin',(57.6,17.3,31.45));
#22665=CARTESIAN_POINT('',(57.6,16.7,31.45));
#22666=CARTESIAN_POINT('Origin',(57.6,17.3,31.45));
#22667=CARTESIAN_POINT('',(57.6,16.7,32.55));
#22668=CARTESIAN_POINT('',(57.6,16.7,31.45));
#22669=CARTESIAN_POINT('Origin',(57.6,17.3,32.55));
#22670=CARTESIAN_POINT('Origin',(52.4,16.7,31.45));
#22671=CARTESIAN_POINT('',(52.4,16.7,31.45));
#22672=CARTESIAN_POINT('',(78.7,16.7,31.45));
#22673=CARTESIAN_POINT('',(52.4,16.7,32.55));
#22674=CARTESIAN_POINT('',(52.4,16.7,31.45));
#22675=CARTESIAN_POINT('',(78.7,16.7,32.55));
#22676=CARTESIAN_POINT('Origin',(52.4,17.3,31.45));
#22677=CARTESIAN_POINT('Origin',(52.4,17.3,31.45));
#22678=CARTESIAN_POINT('Origin',(52.4,17.3,32.55));
#22679=CARTESIAN_POINT('Origin',(71.8,24.7,31.45));
#22680=CARTESIAN_POINT('',(71.8,24.7,31.45));
#22681=CARTESIAN_POINT('',(71.8,17.3,31.45));
#22682=CARTESIAN_POINT('',(71.8,22.85,31.45));
#22683=CARTESIAN_POINT('',(71.8,24.7,32.55));
#22684=CARTESIAN_POINT('',(71.8,24.7,31.45));
#22685=CARTESIAN_POINT('',(71.8,17.3,32.55));
#22686=CARTESIAN_POINT('',(71.8,22.85,32.55));
#22687=CARTESIAN_POINT('',(71.8,17.3,31.45));
#22688=CARTESIAN_POINT('Origin',(72.4,24.7,31.45));
#22689=CARTESIAN_POINT('',(72.4,25.3,31.45));
#22690=CARTESIAN_POINT('Origin',(72.4,24.7,31.45));
#22691=CARTESIAN_POINT('',(72.4,25.3,32.55));
#22692=CARTESIAN_POINT('',(72.4,25.3,31.45));
#22693=CARTESIAN_POINT('Origin',(72.4,24.7,32.55));
#22694=CARTESIAN_POINT('Origin',(77.6,25.3,31.45));
#22695=CARTESIAN_POINT('',(77.6,25.3,31.45));
#22696=CARTESIAN_POINT('',(91.3,25.3,31.45));
#22697=CARTESIAN_POINT('',(77.6,25.3,32.55));
#22698=CARTESIAN_POINT('',(77.6,25.3,31.45));
#22699=CARTESIAN_POINT('',(91.3,25.3,32.55));
#22700=CARTESIAN_POINT('Origin',(77.6,24.7,31.45));
#22701=CARTESIAN_POINT('',(78.2,24.7,31.45));
#22702=CARTESIAN_POINT('Origin',(77.6,24.7,31.45));
#22703=CARTESIAN_POINT('',(78.2,24.7,32.55));
#22704=CARTESIAN_POINT('',(78.2,24.7,31.45));
#22705=CARTESIAN_POINT('Origin',(77.6,24.7,32.55));
#22706=CARTESIAN_POINT('Origin',(78.2,17.3,31.45));
#22707=CARTESIAN_POINT('',(78.2,17.3,31.45));
#22708=CARTESIAN_POINT('',(78.2,19.15,31.45));
#22709=CARTESIAN_POINT('',(78.2,17.3,32.55));
#22710=CARTESIAN_POINT('',(78.2,17.3,31.45));
#22711=CARTESIAN_POINT('',(78.2,19.15,32.55));
#22712=CARTESIAN_POINT('Origin',(77.6,17.3,31.45));
#22713=CARTESIAN_POINT('',(77.6,16.7,31.45));
#22714=CARTESIAN_POINT('Origin',(77.6,17.3,31.45));
#22715=CARTESIAN_POINT('',(77.6,16.7,32.55));
#22716=CARTESIAN_POINT('',(77.6,16.7,31.45));
#22717=CARTESIAN_POINT('Origin',(77.6,17.3,32.55));
#22718=CARTESIAN_POINT('Origin',(72.4,16.7,31.45));
#22719=CARTESIAN_POINT('',(72.4,16.7,31.45));
#22720=CARTESIAN_POINT('',(88.7,16.7,31.45));
#22721=CARTESIAN_POINT('',(72.4,16.7,32.55));
#22722=CARTESIAN_POINT('',(72.4,16.7,31.45));
#22723=CARTESIAN_POINT('',(88.7,16.7,32.55));
#22724=CARTESIAN_POINT('Origin',(72.4,17.3,31.45));
#22725=CARTESIAN_POINT('Origin',(72.4,17.3,31.45));
#22726=CARTESIAN_POINT('Origin',(72.4,17.3,32.55));
#22727=CARTESIAN_POINT('Origin',(91.8,24.7,31.45));
#22728=CARTESIAN_POINT('',(91.8,24.7,31.45));
#22729=CARTESIAN_POINT('',(91.8,17.3,31.45));
#22730=CARTESIAN_POINT('',(91.8,22.85,31.45));
#22731=CARTESIAN_POINT('',(91.8,24.7,32.55));
#22732=CARTESIAN_POINT('',(91.8,24.7,31.45));
#22733=CARTESIAN_POINT('',(91.8,17.3,32.55));
#22734=CARTESIAN_POINT('',(91.8,22.85,32.55));
#22735=CARTESIAN_POINT('',(91.8,17.3,31.45));
#22736=CARTESIAN_POINT('Origin',(92.4,24.7,31.45));
#22737=CARTESIAN_POINT('',(92.4,25.3,31.45));
#22738=CARTESIAN_POINT('Origin',(92.4,24.7,31.45));
#22739=CARTESIAN_POINT('',(92.4,25.3,32.55));
#22740=CARTESIAN_POINT('',(92.4,25.3,31.45));
#22741=CARTESIAN_POINT('Origin',(92.4,24.7,32.55));
#22742=CARTESIAN_POINT('Origin',(97.6,25.3,31.45));
#22743=CARTESIAN_POINT('',(97.6,25.3,31.45));
#22744=CARTESIAN_POINT('',(101.3,25.3,31.45));
#22745=CARTESIAN_POINT('',(97.6,25.3,32.55));
#22746=CARTESIAN_POINT('',(97.6,25.3,31.45));
#22747=CARTESIAN_POINT('',(101.3,25.3,32.55));
#22748=CARTESIAN_POINT('Origin',(97.6,24.7,31.45));
#22749=CARTESIAN_POINT('',(98.2,24.7,31.45));
#22750=CARTESIAN_POINT('Origin',(97.6,24.7,31.45));
#22751=CARTESIAN_POINT('',(98.2,24.7,32.55));
#22752=CARTESIAN_POINT('',(98.2,24.7,31.45));
#22753=CARTESIAN_POINT('Origin',(97.6,24.7,32.55));
#22754=CARTESIAN_POINT('Origin',(98.2,17.3,31.45));
#22755=CARTESIAN_POINT('',(98.2,17.3,31.45));
#22756=CARTESIAN_POINT('',(98.2,19.15,31.45));
#22757=CARTESIAN_POINT('',(98.2,17.3,32.55));
#22758=CARTESIAN_POINT('',(98.2,17.3,31.45));
#22759=CARTESIAN_POINT('',(98.2,19.15,32.55));
#22760=CARTESIAN_POINT('Origin',(97.6,17.3,31.45));
#22761=CARTESIAN_POINT('',(97.6,16.7,31.45));
#22762=CARTESIAN_POINT('Origin',(97.6,17.3,31.45));
#22763=CARTESIAN_POINT('',(97.6,16.7,32.55));
#22764=CARTESIAN_POINT('',(97.6,16.7,31.45));
#22765=CARTESIAN_POINT('Origin',(97.6,17.3,32.55));
#22766=CARTESIAN_POINT('Origin',(92.4,16.7,31.45));
#22767=CARTESIAN_POINT('',(92.4,16.7,31.45));
#22768=CARTESIAN_POINT('',(98.7,16.7,31.45));
#22769=CARTESIAN_POINT('',(92.4,16.7,32.55));
#22770=CARTESIAN_POINT('',(92.4,16.7,31.45));
#22771=CARTESIAN_POINT('',(98.7,16.7,32.55));
#22772=CARTESIAN_POINT('Origin',(92.4,17.3,31.45));
#22773=CARTESIAN_POINT('Origin',(92.4,17.3,31.45));
#22774=CARTESIAN_POINT('Origin',(92.4,17.3,32.55));
#22775=CARTESIAN_POINT('Origin',(41.8,24.7,31.45));
#22776=CARTESIAN_POINT('',(41.8,24.7,31.45));
#22777=CARTESIAN_POINT('',(41.8,17.3,31.45));
#22778=CARTESIAN_POINT('',(41.8,22.85,31.45));
#22779=CARTESIAN_POINT('',(41.8,24.7,32.55));
#22780=CARTESIAN_POINT('',(41.8,24.7,31.45));
#22781=CARTESIAN_POINT('',(41.8,17.3,32.55));
#22782=CARTESIAN_POINT('',(41.8,22.85,32.55));
#22783=CARTESIAN_POINT('',(41.8,17.3,31.45));
#22784=CARTESIAN_POINT('Origin',(42.4,24.7,31.45));
#22785=CARTESIAN_POINT('',(42.4,25.3,31.45));
#22786=CARTESIAN_POINT('Origin',(42.4,24.7,31.45));
#22787=CARTESIAN_POINT('',(42.4,25.3,32.55));
#22788=CARTESIAN_POINT('',(42.4,25.3,31.45));
#22789=CARTESIAN_POINT('Origin',(42.4,24.7,32.55));
#22790=CARTESIAN_POINT('Origin',(47.6,25.3,31.45));
#22791=CARTESIAN_POINT('',(47.6,25.3,31.45));
#22792=CARTESIAN_POINT('',(76.3,25.3,31.45));
#22793=CARTESIAN_POINT('',(47.6,25.3,32.55));
#22794=CARTESIAN_POINT('',(47.6,25.3,31.45));
#22795=CARTESIAN_POINT('',(76.3,25.3,32.55));
#22796=CARTESIAN_POINT('Origin',(47.6,24.7,31.45));
#22797=CARTESIAN_POINT('',(48.2,24.7,31.45));
#22798=CARTESIAN_POINT('Origin',(47.6,24.7,31.45));
#22799=CARTESIAN_POINT('',(48.2,24.7,32.55));
#22800=CARTESIAN_POINT('',(48.2,24.7,31.45));
#22801=CARTESIAN_POINT('Origin',(47.6,24.7,32.55));
#22802=CARTESIAN_POINT('Origin',(48.2,17.3,31.45));
#22803=CARTESIAN_POINT('',(48.2,17.3,31.45));
#22804=CARTESIAN_POINT('',(48.2,19.15,31.45));
#22805=CARTESIAN_POINT('',(48.2,17.3,32.55));
#22806=CARTESIAN_POINT('',(48.2,17.3,31.45));
#22807=CARTESIAN_POINT('',(48.2,19.15,32.55));
#22808=CARTESIAN_POINT('Origin',(47.6,17.3,31.45));
#22809=CARTESIAN_POINT('',(47.6,16.7,31.45));
#22810=CARTESIAN_POINT('Origin',(47.6,17.3,31.45));
#22811=CARTESIAN_POINT('',(47.6,16.7,32.55));
#22812=CARTESIAN_POINT('',(47.6,16.7,31.45));
#22813=CARTESIAN_POINT('Origin',(47.6,17.3,32.55));
#22814=CARTESIAN_POINT('Origin',(42.4,16.7,31.45));
#22815=CARTESIAN_POINT('',(42.4,16.7,31.45));
#22816=CARTESIAN_POINT('',(73.7,16.7,31.45));
#22817=CARTESIAN_POINT('',(42.4,16.7,32.55));
#22818=CARTESIAN_POINT('',(42.4,16.7,31.45));
#22819=CARTESIAN_POINT('',(73.7,16.7,32.55));
#22820=CARTESIAN_POINT('Origin',(42.4,17.3,31.45));
#22821=CARTESIAN_POINT('Origin',(42.4,17.3,31.45));
#22822=CARTESIAN_POINT('Origin',(42.4,17.3,32.55));
#22823=CARTESIAN_POINT('Origin',(121.8,24.7,31.45));
#22824=CARTESIAN_POINT('',(121.8,24.7,31.45));
#22825=CARTESIAN_POINT('',(121.8,17.3,31.45));
#22826=CARTESIAN_POINT('',(121.8,22.85,31.45));
#22827=CARTESIAN_POINT('',(121.8,24.7,32.55));
#22828=CARTESIAN_POINT('',(121.8,24.7,31.45));
#22829=CARTESIAN_POINT('',(121.8,17.3,32.55));
#22830=CARTESIAN_POINT('',(121.8,22.85,32.55));
#22831=CARTESIAN_POINT('',(121.8,17.3,31.45));
#22832=CARTESIAN_POINT('Origin',(122.4,24.7,31.45));
#22833=CARTESIAN_POINT('',(122.4,25.3,31.45));
#22834=CARTESIAN_POINT('Origin',(122.4,24.7,31.45));
#22835=CARTESIAN_POINT('',(122.4,25.3,32.55));
#22836=CARTESIAN_POINT('',(122.4,25.3,31.45));
#22837=CARTESIAN_POINT('Origin',(122.4,24.7,32.55));
#22838=CARTESIAN_POINT('Origin',(127.6,25.3,31.45));
#22839=CARTESIAN_POINT('',(127.6,25.3,31.45));
#22840=CARTESIAN_POINT('',(116.3,25.3,31.45));
#22841=CARTESIAN_POINT('',(127.6,25.3,32.55));
#22842=CARTESIAN_POINT('',(127.6,25.3,31.45));
#22843=CARTESIAN_POINT('',(116.3,25.3,32.55));
#22844=CARTESIAN_POINT('Origin',(127.6,24.7,31.45));
#22845=CARTESIAN_POINT('',(128.2,24.7,31.45));
#22846=CARTESIAN_POINT('Origin',(127.6,24.7,31.45));
#22847=CARTESIAN_POINT('',(128.2,24.7,32.55));
#22848=CARTESIAN_POINT('',(128.2,24.7,31.45));
#22849=CARTESIAN_POINT('Origin',(127.6,24.7,32.55));
#22850=CARTESIAN_POINT('Origin',(128.2,17.3,31.45));
#22851=CARTESIAN_POINT('',(128.2,17.3,31.45));
#22852=CARTESIAN_POINT('',(128.2,19.15,31.45));
#22853=CARTESIAN_POINT('',(128.2,17.3,32.55));
#22854=CARTESIAN_POINT('',(128.2,17.3,31.45));
#22855=CARTESIAN_POINT('',(128.2,19.15,32.55));
#22856=CARTESIAN_POINT('Origin',(127.6,17.3,31.45));
#22857=CARTESIAN_POINT('',(127.6,16.7,31.45));
#22858=CARTESIAN_POINT('Origin',(127.6,17.3,31.45));
#22859=CARTESIAN_POINT('',(127.6,16.7,32.55));
#22860=CARTESIAN_POINT('',(127.6,16.7,31.45));
#22861=CARTESIAN_POINT('Origin',(127.6,17.3,32.55));
#22862=CARTESIAN_POINT('Origin',(122.4,16.7,31.45));
#22863=CARTESIAN_POINT('',(122.4,16.7,31.45));
#22864=CARTESIAN_POINT('',(113.7,16.7,31.45));
#22865=CARTESIAN_POINT('',(122.4,16.7,32.55));
#22866=CARTESIAN_POINT('',(122.4,16.7,31.45));
#22867=CARTESIAN_POINT('',(113.7,16.7,32.55));
#22868=CARTESIAN_POINT('Origin',(122.4,17.3,31.45));
#22869=CARTESIAN_POINT('Origin',(122.4,17.3,31.45));
#22870=CARTESIAN_POINT('Origin',(122.4,17.3,32.55));
#22871=CARTESIAN_POINT('Origin',(141.8,24.7,31.45));
#22872=CARTESIAN_POINT('',(141.8,24.7,31.45));
#22873=CARTESIAN_POINT('',(141.8,17.3,31.45));
#22874=CARTESIAN_POINT('',(141.8,22.85,31.45));
#22875=CARTESIAN_POINT('',(141.8,24.7,32.55));
#22876=CARTESIAN_POINT('',(141.8,24.7,31.45));
#22877=CARTESIAN_POINT('',(141.8,17.3,32.55));
#22878=CARTESIAN_POINT('',(141.8,22.85,32.55));
#22879=CARTESIAN_POINT('',(141.8,17.3,31.45));
#22880=CARTESIAN_POINT('Origin',(142.4,24.7,31.45));
#22881=CARTESIAN_POINT('',(142.4,25.3,31.45));
#22882=CARTESIAN_POINT('Origin',(142.4,24.7,31.45));
#22883=CARTESIAN_POINT('',(142.4,25.3,32.55));
#22884=CARTESIAN_POINT('',(142.4,25.3,31.45));
#22885=CARTESIAN_POINT('Origin',(142.4,24.7,32.55));
#22886=CARTESIAN_POINT('Origin',(147.6,25.3,31.45));
#22887=CARTESIAN_POINT('',(147.6,25.3,31.45));
#22888=CARTESIAN_POINT('',(126.3,25.3,31.45));
#22889=CARTESIAN_POINT('',(147.6,25.3,32.55));
#22890=CARTESIAN_POINT('',(147.6,25.3,31.45));
#22891=CARTESIAN_POINT('',(126.3,25.3,32.55));
#22892=CARTESIAN_POINT('Origin',(147.6,24.7,31.45));
#22893=CARTESIAN_POINT('',(148.2,24.7,31.45));
#22894=CARTESIAN_POINT('Origin',(147.6,24.7,31.45));
#22895=CARTESIAN_POINT('',(148.2,24.7,32.55));
#22896=CARTESIAN_POINT('',(148.2,24.7,31.45));
#22897=CARTESIAN_POINT('Origin',(147.6,24.7,32.55));
#22898=CARTESIAN_POINT('Origin',(148.2,17.3,31.45));
#22899=CARTESIAN_POINT('',(148.2,17.3,31.45));
#22900=CARTESIAN_POINT('',(148.2,19.15,31.45));
#22901=CARTESIAN_POINT('',(148.2,17.3,32.55));
#22902=CARTESIAN_POINT('',(148.2,17.3,31.45));
#22903=CARTESIAN_POINT('',(148.2,19.15,32.55));
#22904=CARTESIAN_POINT('Origin',(147.6,17.3,31.45));
#22905=CARTESIAN_POINT('',(147.6,16.7,31.45));
#22906=CARTESIAN_POINT('Origin',(147.6,17.3,31.45));
#22907=CARTESIAN_POINT('',(147.6,16.7,32.55));
#22908=CARTESIAN_POINT('',(147.6,16.7,31.45));
#22909=CARTESIAN_POINT('Origin',(147.6,17.3,32.55));
#22910=CARTESIAN_POINT('Origin',(142.4,16.7,31.45));
#22911=CARTESIAN_POINT('',(142.4,16.7,31.45));
#22912=CARTESIAN_POINT('',(123.7,16.7,31.45));
#22913=CARTESIAN_POINT('',(142.4,16.7,32.55));
#22914=CARTESIAN_POINT('',(142.4,16.7,31.45));
#22915=CARTESIAN_POINT('',(123.7,16.7,32.55));
#22916=CARTESIAN_POINT('Origin',(142.4,17.3,31.45));
#22917=CARTESIAN_POINT('Origin',(142.4,17.3,31.45));
#22918=CARTESIAN_POINT('Origin',(142.4,17.3,32.55));
#22919=CARTESIAN_POINT('Origin',(161.8,24.7,31.45));
#22920=CARTESIAN_POINT('',(161.8,24.7,31.45));
#22921=CARTESIAN_POINT('',(161.8,17.3,31.45));
#22922=CARTESIAN_POINT('',(161.8,22.85,31.45));
#22923=CARTESIAN_POINT('',(161.8,24.7,32.55));
#22924=CARTESIAN_POINT('',(161.8,24.7,31.45));
#22925=CARTESIAN_POINT('',(161.8,17.3,32.55));
#22926=CARTESIAN_POINT('',(161.8,22.85,32.55));
#22927=CARTESIAN_POINT('',(161.8,17.3,31.45));
#22928=CARTESIAN_POINT('Origin',(162.4,24.7,31.45));
#22929=CARTESIAN_POINT('',(162.4,25.3,31.45));
#22930=CARTESIAN_POINT('Origin',(162.4,24.7,31.45));
#22931=CARTESIAN_POINT('',(162.4,25.3,32.55));
#22932=CARTESIAN_POINT('',(162.4,25.3,31.45));
#22933=CARTESIAN_POINT('Origin',(162.4,24.7,32.55));
#22934=CARTESIAN_POINT('Origin',(167.6,25.3,31.45));
#22935=CARTESIAN_POINT('',(167.6,25.3,31.45));
#22936=CARTESIAN_POINT('',(136.3,25.3,31.45));
#22937=CARTESIAN_POINT('',(167.6,25.3,32.55));
#22938=CARTESIAN_POINT('',(167.6,25.3,31.45));
#22939=CARTESIAN_POINT('',(136.3,25.3,32.55));
#22940=CARTESIAN_POINT('Origin',(167.6,24.7,31.45));
#22941=CARTESIAN_POINT('',(168.2,24.7,31.45));
#22942=CARTESIAN_POINT('Origin',(167.6,24.7,31.45));
#22943=CARTESIAN_POINT('',(168.2,24.7,32.55));
#22944=CARTESIAN_POINT('',(168.2,24.7,31.45));
#22945=CARTESIAN_POINT('Origin',(167.6,24.7,32.55));
#22946=CARTESIAN_POINT('Origin',(168.2,17.3,31.45));
#22947=CARTESIAN_POINT('',(168.2,17.3,31.45));
#22948=CARTESIAN_POINT('',(168.2,19.15,31.45));
#22949=CARTESIAN_POINT('',(168.2,17.3,32.55));
#22950=CARTESIAN_POINT('',(168.2,17.3,31.45));
#22951=CARTESIAN_POINT('',(168.2,19.15,32.55));
#22952=CARTESIAN_POINT('Origin',(167.6,17.3,31.45));
#22953=CARTESIAN_POINT('',(167.6,16.7,31.45));
#22954=CARTESIAN_POINT('Origin',(167.6,17.3,31.45));
#22955=CARTESIAN_POINT('',(167.6,16.7,32.55));
#22956=CARTESIAN_POINT('',(167.6,16.7,31.45));
#22957=CARTESIAN_POINT('Origin',(167.6,17.3,32.55));
#22958=CARTESIAN_POINT('Origin',(162.4,16.7,31.45));
#22959=CARTESIAN_POINT('',(162.4,16.7,31.45));
#22960=CARTESIAN_POINT('',(133.7,16.7,31.45));
#22961=CARTESIAN_POINT('',(162.4,16.7,32.55));
#22962=CARTESIAN_POINT('',(162.4,16.7,31.45));
#22963=CARTESIAN_POINT('',(133.7,16.7,32.55));
#22964=CARTESIAN_POINT('Origin',(162.4,17.3,31.45));
#22965=CARTESIAN_POINT('Origin',(162.4,17.3,31.45));
#22966=CARTESIAN_POINT('Origin',(162.4,17.3,32.55));
#22967=CARTESIAN_POINT('Origin',(39.,32.,31.45));
#22968=CARTESIAN_POINT('',(39.,32.,31.45));
#22969=CARTESIAN_POINT('',(39.,10.,31.45));
#22970=CARTESIAN_POINT('',(39.,32.,31.45));
#22971=CARTESIAN_POINT('',(39.,10.,32.55));
#22972=CARTESIAN_POINT('',(39.,10.,31.45));
#22973=CARTESIAN_POINT('',(39.,32.,32.55));
#22974=CARTESIAN_POINT('',(39.,32.,32.55));
#22975=CARTESIAN_POINT('',(39.,32.,31.45));
#22976=CARTESIAN_POINT('Origin',(40.,32.,31.45));
#22977=CARTESIAN_POINT('',(40.,33.,31.45));
#22978=CARTESIAN_POINT('Origin',(40.,32.,31.45));
#22979=CARTESIAN_POINT('',(40.,33.,32.55));
#22980=CARTESIAN_POINT('Origin',(40.,32.,32.55));
#22981=CARTESIAN_POINT('',(40.,33.,31.45));
#22982=CARTESIAN_POINT('Origin',(170.,33.,31.45));
#22983=CARTESIAN_POINT('',(170.,33.,31.45));
#22984=CARTESIAN_POINT('',(170.,33.,31.45));
#22985=CARTESIAN_POINT('',(170.,33.,32.55));
#22986=CARTESIAN_POINT('',(170.,33.,32.55));
#22987=CARTESIAN_POINT('',(170.,33.,31.45));
#22988=CARTESIAN_POINT('Origin',(170.,32.,31.45));
#22989=CARTESIAN_POINT('',(171.,32.,31.45));
#22990=CARTESIAN_POINT('Origin',(170.,32.,31.45));
#22991=CARTESIAN_POINT('',(171.,32.,32.55));
#22992=CARTESIAN_POINT('Origin',(170.,32.,32.55));
#22993=CARTESIAN_POINT('',(171.,32.,31.45));
#22994=CARTESIAN_POINT('Origin',(171.,10.,31.45));
#22995=CARTESIAN_POINT('',(171.,10.,31.45));
#22996=CARTESIAN_POINT('',(171.,10.,31.45));
#22997=CARTESIAN_POINT('',(171.,10.,32.55));
#22998=CARTESIAN_POINT('',(171.,10.,32.55));
#22999=CARTESIAN_POINT('',(171.,10.,31.45));
#23000=CARTESIAN_POINT('Origin',(170.,10.,31.45));
#23001=CARTESIAN_POINT('',(170.,9.,31.45));
#23002=CARTESIAN_POINT('Origin',(170.,10.,31.45));
#23003=CARTESIAN_POINT('',(170.,9.,32.55));
#23004=CARTESIAN_POINT('Origin',(170.,10.,32.55));
#23005=CARTESIAN_POINT('',(170.,9.,31.45));
#23006=CARTESIAN_POINT('Origin',(40.,9.,31.45));
#23007=CARTESIAN_POINT('',(40.,9.,31.45));
#23008=CARTESIAN_POINT('',(40.,9.,31.45));
#23009=CARTESIAN_POINT('',(40.,9.,32.55));
#23010=CARTESIAN_POINT('',(40.,9.,32.55));
#23011=CARTESIAN_POINT('',(40.,9.,31.45));
#23012=CARTESIAN_POINT('Origin',(40.,10.,31.45));
#23013=CARTESIAN_POINT('Origin',(40.,10.,31.45));
#23014=CARTESIAN_POINT('Origin',(40.,10.,32.55));
#23015=CARTESIAN_POINT('Origin',(105.,21.,32.55));
#23016=CARTESIAN_POINT('Origin',(105.,21.,31.45));
#81022=UNCERTAINTY_MEASURE_WITH_UNIT(LENGTH_MEASURE(0.01),#81041,
'DISTANCE_ACCURACY_VALUE',
'Maximum model space distance between geometric entities at asserted c
onnectivities');
#81028=UNCERTAINTY_MEASURE_WITH_UNIT(LENGTH_MEASURE(0.01),#81041,
'DISTANCE_ACCURACY_VALUE',
'Maximum model space distance between geometric entities at asserted c
onnectivities');
#81034=(
GEOMETRIC_REPRESENTATION_CONTEXT(3)
GLOBAL_UNCERTAINTY_ASSIGNED_CONTEXT((#81022))
GLOBAL_UNIT_ASSIGNED_CONTEXT((#81041,#81043,#81044))
REPRESENTATION_CONTEXT('','3D')
);
#81040=(
GEOMETRIC_REPRESENTATION_CONTEXT(3)
GLOBAL_UNCERTAINTY_ASSIGNED_CONTEXT((#81028))
GLOBAL_UNIT_ASSIGNED_CONTEXT((#81041,#81043,#81044))
REPRESENTATION_CONTEXT('','3D')
);
#81041=(
LENGTH_UNIT()
NAMED_UNIT(*)
SI_UNIT(.MILLI.,.METRE.)
);
#81043=(
NAMED_UNIT(*)
PLANE_ANGLE_UNIT()
SI_UNIT($,.RADIAN.)
);
#81044=(
NAMED_UNIT(*)
SI_UNIT($,.STERADIAN.)
SOLID_ANGLE_UNIT()
);
#81050=SHAPE_DEFINITION_REPRESENTATION(#81061,#81134);
#81061=PRODUCT_DEFINITION_SHAPE('',$,#81146);
#81134=SHAPE_REPRESENTATION('',(#15816),#81034);
#81140=PRODUCT_DEFINITION_CONTEXT('part definition',#81175,'design');
#81146=PRODUCT_DEFINITION('Cross-Roller Cage Strip',
'Cross-Roller Cage Strip',#81157,#81140);
#81157=PRODUCT_DEFINITION_FORMATION('',$,#81182);
#81175=APPLICATION_CONTEXT(
'Core Data for Automotive Mechanical Design Process');
#81176=PRODUCT_CONTEXT('part definition',#81175,'mechanical');
#81182=PRODUCT('Cross-Roller Cage Strip','Cross-Roller Cage Strip',$,(#81176));
#81193=PRESENTATION_STYLE_ASSIGNMENT((#81204));
#81204=SURFACE_STYLE_USAGE(.BOTH.,#81215);
#81215=SURFACE_SIDE_STYLE('',(#81226));
#81226=SURFACE_STYLE_FILL_AREA(#81237);
#81237=FILL_AREA_STYLE('Opaque(194,198,204)',(#81248));
#81248=FILL_AREA_STYLE_COLOUR('Opaque(194,198,204)',#81259);
#81259=COLOUR_RGB('Opaque(194,198,204)', 0.72549020, 0.75294118, 0.79215686);
ENDSEC;
END-ISO-10303-21;
